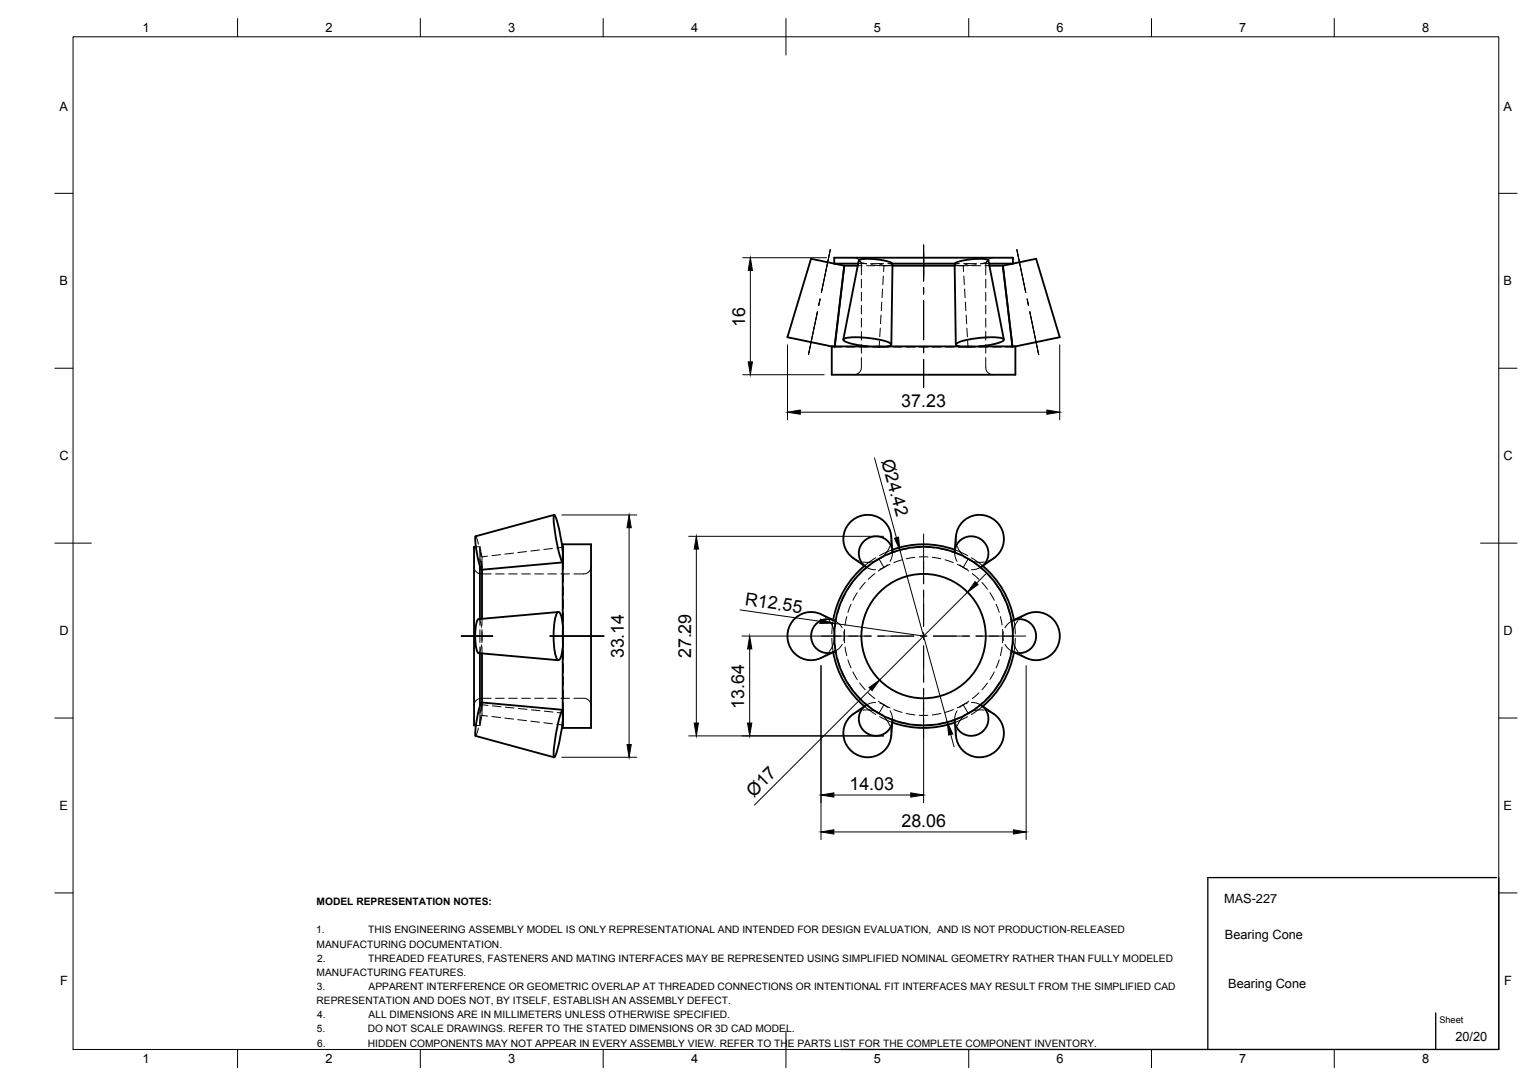
ISO-10303-21;
HEADER;
FILE_DESCRIPTION (('STEP AP214'),
    '1' );
FILE_NAME ( 'Bearing Cone.step', '2026-10-06T08:24:41', ( '' ), ( '' ), 'STEP AP214', 'Unspecified', '' );
FILE_SCHEMA (( 'AUTOMOTIVE_DESIGN' ));
ENDSEC;
DATA;
#68=CARTESIAN_POINT ( 'NONE',  ( 0.1516263115863346334, -0.2937912646890007973, 0.3972688187320929099 ) ) ;
#70=FACE_OUTER_BOUND ( 'NONE', #14571, .T. ) ;
#91=CYLINDRICAL_SURFACE ( 'NONE', #13414, 0.4941010236220472751 ) ;
#116=EDGE_LOOP ( 'NONE', ( #3270, #475, #22588, #2347 ) ) ;
#150=ADVANCED_FACE ( 'NONE', ( #5405 ), #14023, .T. ) ;
#166=CARTESIAN_POINT ( 'NONE',  ( 0.1490609433494345659, -0.2352065284464384953, -0.4168512521180542385 ) ) ;
#181=( BOUNDED_CURVE ( )  B_SPLINE_CURVE ( 3, ( #15130, #19634, #17231, #21476 ),
 .UNSPECIFIED., .F., .F. ) 
 B_SPLINE_CURVE_WITH_KNOTS ( ( 4, 4 ),
 ( 6.170019055269735375, 6.396351559089437089 ),
 .UNSPECIFIED. ) 
 CURVE ( )  GEOMETRIC_REPRESENTATION_ITEM ( )  RATIONAL_B_SPLINE_CURVE ( ( 1.000000000000000000, 0.9957356870045847019, 0.9957356870045847019, 1.000000000000000000 ) ) 
 REPRESENTATION_ITEM ( '' )  ) ;
#206=DIRECTION ( 'NONE',  ( 0.000000000000000000, 1.000000000000000000, 0.000000000000000000 ) ) ;
#228=ORIENTED_EDGE ( 'NONE', *, *, #21922, .T. ) ;
#246=CARTESIAN_POINT ( 'NONE',  ( 0.1490609433615242285, 0.4786070381542913421, 0.000000000000000000 ) ) ;
#280=VERTEX_POINT ( 'NONE', #5695 ) ;
#284=EDGE_CURVE ( 'NONE', #11054, #21365, #5605, .T. ) ;
#304=B_SPLINE_CURVE_WITH_KNOTS ( 'NONE', 3,
 ( #11360, #4990, #21548, #4455 ),
 .UNSPECIFIED., .F., .F.,
 ( 4, 4 ),
 ( 1.743059029969425078, 1.744705333033724992 ),
 .UNSPECIFIED. ) ;
#356=ADVANCED_FACE ( 'NONE', ( #15159 ), #8639, .T. ) ;
#373=EDGE_CURVE ( 'NONE', #24937, #5795, #15104, .T. ) ;
#380=EDGE_CURVE ( 'NONE', #22824, #12297, #25600, .T. ) ;
#390=AXIS2_PLACEMENT_3D ( 'NONE', #12393, #16488, #25245 ) ;
#413=ORIENTED_EDGE ( 'NONE', *, *, #20952, .T. ) ;
#463=ORIENTED_EDGE ( 'NONE', *, *, #26682, .F. ) ;
#468=CARTESIAN_POINT ( 'NONE',  ( 0.1525037638700916243, 0.2314035372547586233, -0.4381595109572587465 ) ) ;
#475=ORIENTED_EDGE ( 'NONE', *, *, #3137, .F. ) ;
#498=DIRECTION ( 'NONE',  ( 0.000000000000000000, 1.000000000000000000, 0.000000000000000000 ) ) ;
#503=LINE ( 'NONE', #20402, #13869 ) ;
#519=FACE_OUTER_BOUND ( 'NONE', #10794, .T. ) ;
#524=LINE ( 'NONE', #2219, #4201 ) ;
#525=CARTESIAN_POINT ( 'NONE',  ( 0.1490609433494345937, 0.2434005097105403082, -0.4121204548294903347 ) ) ;
#532=B_SPLINE_CURVE_WITH_KNOTS ( 'NONE', 3,
 ( #24989, #10725, #23173, #16808 ),
 .UNSPECIFIED., .F., .F.,
 ( 4, 4 ),
 ( 0.9895101543494979612, 0.9911564574137969874 ),
 .UNSPECIFIED. ) ;
#546=DIRECTION ( 'NONE',  ( 1.000000000000000000, 0.000000000000000000, 0.000000000000000000 ) ) ;
#558=DIRECTION ( 'NONE',  ( 1.000000000000000000, 0.000000000000000000, 0.000000000000000000 ) ) ;
#563=ORIENTED_EDGE ( 'NONE', *, *, #5290, .F. ) ;
#593=CARTESIAN_POINT ( 'NONE',  ( 0.2019525613798653918, -0.3664466487725785426, 0.6347042139374529102 ) ) ;
#615=EDGE_CURVE ( 'NONE', #12438, #5795, #14823, .T. ) ;
#627=EDGE_LOOP ( 'NONE', ( #9029, #26205 ) ) ;
#662=ORIENTED_EDGE ( 'NONE', *, *, #19173, .T. ) ;
#665=EDGE_CURVE ( 'NONE', #15651, #12947, #18212, .T. ) ;
#677=AXIS2_PLACEMENT_3D ( 'NONE', #5334, #26801, #20450 ) ;
#679=CARTESIAN_POINT ( 'NONE',  ( 0.1512834625131836974, 0.2028719039650156708, -0.4452748529150018508 ) ) ;
#688=FACE_OUTER_BOUND ( 'NONE', #8896, .T. ) ;
#707=DIRECTION ( 'NONE',  ( 1.000000000000000000, 0.000000000000000000, 0.000000000000000000 ) ) ;
#714=DIRECTION ( 'NONE',  ( -0.9575713608335526539, 0.1440981340193007720, -0.2495852893972995146 ) ) ;
#732=ORIENTED_EDGE ( 'NONE', *, *, #14585, .T. ) ;
#748=CARTESIAN_POINT ( 'NONE',  ( 0.1638952246732497953, 0.5499255957412874096, 0.000000000000000000 ) ) ;
#773=CARTESIAN_POINT ( 'NONE',  ( 0.1493402947442837025, 0.2231667116155127972, 0.4250100353273641440 ) ) ;
#781=DIRECTION ( 'NONE',  ( 0.000000000000000000, -0.8660254037844389297, -0.4999999999999994449 ) ) ;
#807=EDGE_CURVE ( 'NONE', #21046, #2655, #23735, .T. ) ;
#826=CIRCLE ( 'NONE', #11202, 0.1298643763538141760 ) ;
#843=DIRECTION ( 'NONE',  ( -0.9790454724845840673, 0.1018208755700876073, -0.1763589297585415050 ) ) ;
#872=ORIENTED_EDGE ( 'NONE', *, *, #24132, .F. ) ;
#873=AXIS2_PLACEMENT_3D ( 'NONE', #26941, #1100, #24946 ) ;
#898=DIRECTION ( 'NONE',  ( -0.9790454724845842893, -0.1018208755700884260, -0.1763589297585410332 ) ) ;
#904=( CONVERSION_BASED_UNIT ( 'INCH', #18242 ) LENGTH_UNIT ( ) NAMED_UNIT ( #24418 ) ) ;
#907=CARTESIAN_POINT ( 'NONE',  ( 0.6299212598425196763, -0.4807043897637795493, 5.886930922602943265E-17 ) ) ;
#915=CARTESIAN_POINT ( 'NONE',  ( 0.1755067523729419432, -0.3028750839302634112, 0.5245950337139047015 ) ) ;
#983=EDGE_LOOP ( 'NONE', ( #23970, #6463, #1289, #16251, #21520, #7050 ) ) ;
#984=CARTESIAN_POINT ( 'NONE',  ( 0.5869493968219645641, 0.2133897621573078718, 0.3696019098714952711 ) ) ;
#1004=CARTESIAN_POINT ( 'NONE',  ( 0.1490609433494345659, -0.4786070381568058862, -0.004730797288060355210 ) ) ;
#1011=VERTEX_POINT ( 'NONE', #5046 ) ;
#1060=DIRECTION ( 'NONE',  ( 1.000000000000000000, 0.000000000000000000, 0.000000000000000000 ) ) ;
#1100=DIRECTION ( 'NONE',  ( 0.9790454724845839563, -0.2036417511401769909, 0.000000000000000000 ) ) ;
#1114=AXIS2_PLACEMENT_3D ( 'NONE', #7079, #15697, #24300 ) ;
#1125=ORIENTED_EDGE ( 'NONE', *, *, #21190, .F. ) ;
#1130=CARTESIAN_POINT ( 'NONE',  ( 0.1516263115863346334, 0.4909405214979283838, 0.05579628926458630317 ) ) ;
#1146=CARTESIAN_POINT ( 'NONE',  ( 0.1512183756280983948, -0.4867863319339438277, -0.04701115990130280697 ) ) ;
#1151=DIRECTION ( 'NONE',  ( 0.000000000000000000, -1.000000000000000000, 0.000000000000000000 ) ) ;
#1158=CIRCLE ( 'NONE', #19655, 0.3740157480314960647 ) ;
#1186=EDGE_CURVE ( 'NONE', #12297, #1011, #18232, .T. ) ;
#1189=DIRECTION ( 'NONE',  ( -0.9790454724845842893, 0.2036417511401760472, 0.000000000000000000 ) ) ;
#1202=DIRECTION ( 'NONE',  ( 0.000000000000000000, 1.000000000000000000, 0.000000000000000000 ) ) ;
#1209=ORIENTED_EDGE ( 'NONE', *, *, #27427, .F. ) ;
#1231=VERTEX_POINT ( 'NONE', #23141 ) ;
#1241=CARTESIAN_POINT ( 'NONE',  ( 0.1516263115863346334, -0.1971492568089275588, -0.4530651079966787620 ) ) ;
#1262=CONICAL_SURFACE ( 'NONE', #22899, 0.4526932812344527379, 0.1178097243749990780 ) ;
#1265=ORIENTED_EDGE ( 'NONE', *, *, #26244, .T. ) ;
#1275=CARTESIAN_POINT ( 'NONE',  ( 0.1755067523729419432, 0.3028750839302634112, -0.5245950337139054787 ) ) ;
#1276=CIRCLE ( 'NONE', #19786, 0.3346456692913385988 ) ;
#1288=CARTESIAN_POINT ( 'NONE',  ( 0.1522836969735571200, 0.4941010236220468865, 0.01864847287710773294 ) ) ;
#1289=ORIENTED_EDGE ( 'NONE', *, *, #12310, .T. ) ;
#1294=AXIS2_PLACEMENT_3D ( 'NONE', #5908, #12769, #14538 ) ;
#1330=CARTESIAN_POINT ( 'NONE',  ( 0.1501355178992943573, -0.2698857342899688705, -0.4015219628616845671 ) ) ;
#1372=ORIENTED_EDGE ( 'NONE', *, *, #10616, .F. ) ;
#1455=DIRECTION ( 'NONE',  ( 1.000000000000000000, 0.000000000000000000, 0.000000000000000000 ) ) ;
#1592=CARTESIAN_POINT ( 'NONE',  ( 0.1516263115863346334, -0.4909405214979283838, 0.05579628926458630317 ) ) ;
#1605=DIRECTION ( 'NONE',  ( 1.000000000000000000, 0.000000000000000000, 0.000000000000000000 ) ) ;
#1606=B_SPLINE_CURVE_WITH_KNOTS ( 'NONE', 3,
 ( #13341, #17306, #19706, #24214 ),
 .UNSPECIFIED., .F., .F.,
 ( 4, 4 ),
 ( 1.743059029969425078, 1.744705333033724992 ),
 .UNSPECIFIED. ) ;
#1639=CARTESIAN_POINT ( 'NONE',  ( 0.6241887519799540485, -0.3029073140874564696, -0.5246508579836981490 ) ) ;
#1650=ORIENTED_EDGE ( 'NONE', *, *, #22521, .F. ) ;
#1658=DIRECTION ( 'NONE',  ( 0.000000000000000000, 0.000000000000000000, 1.000000000000000000 ) ) ;
#1670=ORIENTED_EDGE ( 'NONE', *, *, #22246, .T. ) ;
#1682=ORIENTED_EDGE ( 'NONE', *, *, #380, .T. ) ;
#1684=CARTESIAN_POINT ( 'NONE',  ( 0.1490609433537086470, -0.2477132731973591961, 0.4096304796931519165 ) ) ;
#1706=FACE_OUTER_BOUND ( 'NONE', #25350, .T. ) ;
#1707=AXIS2_PLACEMENT_3D ( 'NONE', #18329, #15682, #15955 ) ;
#1710=CIRCLE ( 'NONE', #390, 0.09143349766193344108 ) ;
#1722=ORIENTED_EDGE ( 'NONE', *, *, #4721, .T. ) ;
#1723=CARTESIAN_POINT ( 'NONE',  ( 0.1525037638700915965, -0.2314035372547590119, 0.4381595109572582469 ) ) ;
#1725=ORIENTED_EDGE ( 'NONE', *, *, #4241, .T. ) ;
#1752=ADVANCED_FACE ( 'NONE', ( #9783 ), #14715, .T. ) ;
#1760=EDGE_LOOP ( 'NONE', ( #17994, #18349, #7720, #19973 ) ) ;
#1761=CARTESIAN_POINT ( 'NONE',  ( 0.5925575908939920700, 0.000000000000000000, 0.000000000000000000 ) ) ;
#1791=CARTESIAN_POINT ( 'NONE',  ( 0.1490609433615242285, -0.4786070381542913421, 5.861244094488189820E-17 ) ) ;
#1802=VERTEX_POINT ( 'NONE', #20523 ) ;
#1810=ORIENTED_EDGE ( 'NONE', *, *, #27252, .F. ) ;
#1828=CARTESIAN_POINT ( 'NONE',  ( 0.03937007874015747977, 0.000000000000000000, -0.3740157480314960647 ) ) ;
#1832=DIRECTION ( 'NONE',  ( -0.9930684569432060016, -0.1175373975568611284, 1.439417707043116609E-17 ) ) ;
#1851=SURFACE_STYLE_FILL_AREA ( #5675 ) ;
#1889=EDGE_CURVE ( 'NONE', #18210, #12438, #181, .T. ) ;
#1893=CIRCLE ( 'NONE', #7287, 0.09143349766193344108 ) ;
#1908=AXIS2_PLACEMENT_3D ( 'NONE', #8443, #25400, #25959 ) ;
#1917=LINE ( 'NONE', #25369, #23538 ) ;
#1933=AXIS2_PLACEMENT_3D ( 'NONE', #3288, #11638, #1202 ) ;
#1998=DIRECTION ( 'NONE',  ( -0.9790454724845842893, -0.1018208755700880375, -0.1763589297585410332 ) ) ;
#2036=AXIS2_PLACEMENT_3D ( 'NONE', #3197, #18743, #11830 ) ;
#2068=EDGE_LOOP ( 'NONE', ( #14115, #15701, #8761 ) ) ;
#2072=ORIENTED_EDGE ( 'NONE', *, *, #18545, .F. ) ;
#2115=EDGE_CURVE ( 'NONE', #20796, #18835, #23260, .T. ) ;
#2127=ORIENTED_EDGE ( 'NONE', *, *, #27252, .T. ) ;
#2137=CARTESIAN_POINT ( 'NONE',  ( 0.6241887519799541595, 0.3029073140874564696, 0.5246508579836981490 ) ) ;
#2151=EDGE_LOOP ( 'NONE', ( #12416, #19888, #24371, #19139 ) ) ;
#2195=EDGE_CURVE ( 'NONE', #19740, #12947, #25112, .T. ) ;
#2202=DIRECTION ( 'NONE',  ( 0.000000000000000000, -1.000000000000000000, 0.000000000000000000 ) ) ;
#2205=EDGE_LOOP ( 'NONE', ( #5369, #6270, #18830, #662 ) ) ;
#2208=CARTESIAN_POINT ( 'NONE',  ( 0.3680051700917442714, -0.2263466406172265633, -0.3920438816715692831 ) ) ;
#2219=CARTESIAN_POINT ( 'NONE',  ( 0.5869493968219645641, -0.2133897621573078718, -0.3696019098714952711 ) ) ;
#2254=ORIENTED_EDGE ( 'NONE', *, *, #24577, .T. ) ;
#2256=CARTESIAN_POINT ( 'NONE',  ( 0.6241887519799541595, -0.6058146281749130502, 6.299353404003403643E-17 ) ) ;
#2264=ADVANCED_FACE ( 'NONE', ( #19133 ), #3370, .T. ) ;
#2270=CARTESIAN_POINT ( 'NONE',  ( 0.03937007874015747977, 0.000000000000000000, 0.000000000000000000 ) ) ;
#2278=EDGE_CURVE ( 'NONE', #15470, #23305, #13037, .T. ) ;
#2291=CARTESIAN_POINT ( 'NONE',  ( 0.3905379133858267737, 0.2805118110236220486, -0.4858607088160732390 ) ) ;
#2309=ORIENTED_EDGE ( 'NONE', *, *, #20542, .F. ) ;
#2347=ORIENTED_EDGE ( 'NONE', *, *, #4905, .T. ) ;
#2404=CARTESIAN_POINT ( 'NONE',  ( 0.1755067523729419432, -0.3028750839302637998, -0.5245950337139047015 ) ) ;
#2413=AXIS2_PLACEMENT_3D ( 'NONE', #22706, #7306, #5180 ) ;
#2417=ORIENTED_EDGE ( 'NONE', *, *, #4375, .T. ) ;
#2420=EDGE_LOOP ( 'NONE', ( #19438, #3974, #22960, #23219, #17211, #4913 ) ) ;
#2455=DIRECTION ( 'NONE',  ( 0.000000000000000000, 1.000000000000000000, 0.000000000000000000 ) ) ;
#2459=ORIENTED_EDGE ( 'NONE', *, *, #8343, .F. ) ;
#2510=AXIS2_PLACEMENT_3D ( 'NONE', #1761, #15064, #23256 ) ;
#2518=ADVANCED_FACE ( 'NONE', ( #17695 ), #26322, .T. ) ;
#2553=DIRECTION ( 'NONE',  ( -0.2036417511401758251, 0.9790454724845842893, -1.198984999999999602E-16 ) ) ;
#2558=CARTESIAN_POINT ( 'NONE',  ( 0.5869493968219645641, 0.2133897621573074832, -0.3696019098714952711 ) ) ;
#2560=CARTESIAN_POINT ( 'NONE',  ( 0.1525037638700915965, 0.2637554987713723320, -0.4194810972668293614 ) ) ;
#2593=CONICAL_SURFACE ( 'NONE', #18365, 0.4863540308881693086, 1.365720138124999927 ) ;
#2597=EDGE_CURVE ( 'NONE', #27102, #1802, #532, .T. ) ;
#2612=CIRCLE ( 'NONE', #6255, 0.4807043897637795493 ) ;
#2624=CARTESIAN_POINT ( 'NONE',  ( 0.1755067523729419432, -0.3028750839302634112, 0.5245950337139047015 ) ) ;
#2625=DIRECTION ( 'NONE',  ( -0.9790454724845842893, -0.2036417511401760472, 2.493892000000000781E-17 ) ) ;
#2629=VECTOR ( 'NONE', #24396, 39.37007874015748854 ) ;
#2634=EDGE_LOOP ( 'NONE', ( #21709, #12483, #8120, #17743, #16275, #6478 ) ) ;
#2644=CARTESIAN_POINT ( 'NONE',  ( 0.1638952246732497953, 0.2749627978706433162, -0.4762495361032464958 ) ) ;
#2655=VERTEX_POINT ( 'NONE', #1791 ) ;
#2664=LINE ( 'NONE', #17778, #15369 ) ;
#2697=ORIENTED_EDGE ( 'NONE', *, *, #12178, .T. ) ;
#2736=CARTESIAN_POINT ( 'NONE',  ( 0.1493472610806836076, 0.2566546340585424968, 0.4057060197093078080 ) ) ;
#2773=CARTESIAN_POINT ( 'NONE',  ( 0.1490609433615242285, 0.2393035190771452825, -0.4144858534716441278 ) ) ;
#2783=VECTOR ( 'NONE', #20849, 39.37007874015748854 ) ;
#2798=DIRECTION ( 'NONE',  ( -0.2036417511401761582, 0.4895227362422917006, -0.8478782506317886769 ) ) ;
#2800=CARTESIAN_POINT ( 'NONE',  ( 0.1516263115863346334, 0.4909405214979283838, 0.05579628926458630317 ) ) ;
#2815=CIRCLE ( 'NONE', #9598, 0.1298643763538142593 ) ;
#2816=EDGE_CURVE ( 'NONE', #23841, #11054, #503, .T. ) ;
#2818=CARTESIAN_POINT ( 'NONE',  ( 0.4130706566799093316, 0.3346769814300175616, 0.5796775359605756961 ) ) ;
#2821=FACE_OUTER_BOUND ( 'NONE', #2634, .T. ) ;
#2852=ORIENTED_EDGE ( 'NONE', *, *, #10985, .F. ) ;
#2861=DIRECTION ( 'NONE',  ( 0.000000000000000000, -1.000000000000000000, 0.000000000000000000 ) ) ;
#2863=DIRECTION ( 'NONE',  ( 0.000000000000000000, 1.000000000000000000, 0.000000000000000000 ) ) ;
#2893=CARTESIAN_POINT ( 'NONE',  ( 0.1516263115863346334, -0.4909405214979283838, -0.05579628926458622684 ) ) ;
#2912=ADVANCED_FACE ( 'NONE', ( #18261 ), #1262, .T. ) ;
#2942=ADVANCED_FACE ( 'NONE', ( #13763 ), #19849, .T. ) ;
#2964=AXIS2_PLACEMENT_3D ( 'NONE', #20804, #14767, #7960 ) ;
#2969=EDGE_CURVE ( 'NONE', #12210, #21566, #5764, .T. ) ;
#2982=AXIS2_PLACEMENT_3D ( 'NONE', #6922, #558, #9155 ) ;
#2988=DIRECTION ( 'NONE',  ( 1.000000000000000000, 0.000000000000000000, 0.000000000000000000 ) ) ;
#3015=DIRECTION ( 'NONE',  ( 0.2036417511401769631, -0.9790454724845838452, 1.198984999999999849E-16 ) ) ;
#3019=B_SPLINE_CURVE_WITH_KNOTS ( 'NONE', 3,
 ( #8186, #25271, #26975, #1130 ),
 .UNSPECIFIED., .F., .F.,
 ( 4, 4 ),
 ( 0.9893485554301200136, 0.9909948584944189287 ),
 .UNSPECIFIED. ) ;
#3048=FACE_OUTER_BOUND ( 'NONE', #23019, .T. ) ;
#3072=DIRECTION ( 'NONE',  ( -0.9790454724845842893, -0.1018208755700880375, 0.1763589297585410332 ) ) ;
#3137=EDGE_CURVE ( 'NONE', #21046, #13737, #4429, .T. ) ;
#3148=EDGE_LOOP ( 'NONE', ( #27180, #1682, #9509, #8478, #4115, #23919 ) ) ;
#3155=DIRECTION ( 'NONE',  ( -1.000000000000000000, 0.000000000000000000, 0.000000000000000000 ) ) ;
#3158=ORIENTED_EDGE ( 'NONE', *, *, #8802, .T. ) ;
#3164=CARTESIAN_POINT ( 'NONE',  ( 0.6055690743987126590, 0.2581485381169802973, 0.4471263839182408883 ) ) ;
#3170=EDGE_CURVE ( 'NONE', #22329, #8047, #3984, .T. ) ;
#3171=ORIENTED_EDGE ( 'NONE', *, *, #3875, .F. ) ;
#3187=CIRCLE ( 'NONE', #25763, 0.09143349766193348271 ) ;
#3197=CARTESIAN_POINT ( 'NONE',  ( 0.1506723201675407575, 0.000000000000000000, 0.000000000000000000 ) ) ;
#3203=CARTESIAN_POINT ( 'NONE',  ( 0.3149606299212598381, 0.3346456692913385988, 0.000000000000000000 ) ) ;
#3218=DIRECTION ( 'NONE',  ( -0.9790454724845842893, -0.1018208755700880375, 0.1763589297585410332 ) ) ;
#3219=VECTOR ( 'NONE', #21211, 39.37007874015748143 ) ;
#3228=ADVANCED_FACE ( 'NONE', ( #5573 ), #19299, .T. ) ;
#3250=CARTESIAN_POINT ( 'NONE',  ( 0.3905379133858267737, -0.2805118110236220486, 0.4858607088160724063 ) ) ;
#3263=CARTESIAN_POINT ( 'NONE',  ( 0.1522836969735571200, -0.4941010236220468865, 0.01864847287710767396 ) ) ;
#3266=DIRECTION ( 'NONE',  ( -0.2036417511401763802, 0.4895227362422922557, 0.8478782506317883438 ) ) ;
#3270=ORIENTED_EDGE ( 'NONE', *, *, #16719, .F. ) ;
#3283=CARTESIAN_POINT ( 'NONE',  ( 0.1504366439317612048, -0.2089021884548363517, 0.4380456861425212622 ) ) ;
#3286=DIRECTION ( 'NONE',  ( 1.000000000000000000, 0.000000000000000000, 0.000000000000000000 ) ) ;
#3288=CARTESIAN_POINT ( 'NONE',  ( 0.6299212598425196763, 0.4076750295275590741, 0.000000000000000000 ) ) ;
#3316=ORIENTED_EDGE ( 'NONE', *, *, #25771, .F. ) ;
#3331=DIRECTION ( 'NONE',  ( 1.000000000000000000, 0.000000000000000000, 0.000000000000000000 ) ) ;
#3335=ORIENTED_EDGE ( 'NONE', *, *, #7386, .T. ) ;
#3348=EDGE_LOOP ( 'NONE', ( #21676, #27774, #19131, #2459, #17124, #23248 ) ) ;
#3359=EDGE_CURVE ( 'NONE', #24341, #18758, #1276, .T. ) ;
#3370=CONICAL_SURFACE ( 'NONE', #2510, 0.4537419570391968415, 1.365720138124999927 ) ;
#3389=ORIENTED_EDGE ( 'NONE', *, *, #2969, .F. ) ;
#3402=CIRCLE ( 'NONE', #20119, 0.4807043897637795493 ) ;
#3427=DIRECTION ( 'NONE',  ( -0.9790454724845842893, 0.1018208755700882318, 0.1763589297585410332 ) ) ;
#3437=ORIENTED_EDGE ( 'NONE', *, *, #14859, .F. ) ;
#3485=ORIENTED_EDGE ( 'NONE', *, *, #3359, .T. ) ;
#3490=CARTESIAN_POINT ( 'NONE',  ( 0.1512834625133127053, -0.4870552862737996813, 0.04694520391073944698 ) ) ;
#3496=( GEOMETRIC_REPRESENTATION_CONTEXT ( 3 ) GLOBAL_UNCERTAINTY_ASSIGNED_CONTEXT ( ( #12494 ) ) GLOBAL_UNIT_ASSIGNED_CONTEXT ( ( #904, #22221, #26589 ) ) REPRESENTATION_CONTEXT ( 'NONE', 'WORKASPACE' ) ) ;
#3507=DIRECTION ( 'NONE',  ( 1.000000000000000000, 0.000000000000000000, 0.000000000000000000 ) ) ;
#3528=EDGE_CURVE ( 'NONE', #21046, #23841, #15047, .T. ) ;
#3641=EDGE_CURVE ( 'NONE', #23196, #17206, #10923, .T. ) ;
#3647=ORIENTED_EDGE ( 'NONE', *, *, #5093, .T. ) ;
#3707=ORIENTED_EDGE ( 'NONE', *, *, #4905, .F. ) ;
#3712=LINE ( 'NONE', #25184, #26502 ) ;
#3715=DIRECTION ( 'NONE',  ( 0.000000000000000000, 1.000000000000000000, 0.000000000000000000 ) ) ;
#3719=AXIS2_PLACEMENT_3D ( 'NONE', #15864, #10941, #19566 ) ;
#3721=CARTESIAN_POINT ( 'NONE',  ( 0.1516263115863346334, 0.4909405214979283838, -0.05579628926458630317 ) ) ;
#3752=VERTEX_POINT ( 'NONE', #11747 ) ;
#3795=ORIENTED_EDGE ( 'NONE', *, *, #16719, .T. ) ;
#3816=ORIENTED_EDGE ( 'NONE', *, *, #7420, .T. ) ;
#3875=EDGE_CURVE ( 'NONE', #5524, #15921, #14518, .T. ) ;
#3895=AXIS2_PLACEMENT_3D ( 'NONE', #12443, #1151, #14003 ) ;
#3901=AXIS2_PLACEMENT_3D ( 'NONE', #22366, #2988, #20243 ) ;
#3909=CARTESIAN_POINT ( 'NONE',  ( 0.1520645003680120011, -0.1970746732787106437, -0.4530975572029189435 ) ) ;
#3914=ORIENTED_EDGE ( 'NONE', *, *, #13598, .F. ) ;
#3926=ORIENTED_EDGE ( 'NONE', *, *, #25191, .F. ) ;
#3927=DIRECTION ( 'NONE',  ( -1.000000000000000000, 0.000000000000000000, 0.000000000000000000 ) ) ;
#3949=CARTESIAN_POINT ( 'NONE',  ( 0.1491281042588008532, -0.2312610231601890387, -0.4194211939771484432 ) ) ;
#3961=ORIENTED_EDGE ( 'NONE', *, *, #5628, .T. ) ;
#3964=EDGE_CURVE ( 'NONE', #19596, #7184, #4695, .T. ) ;
#3974=ORIENTED_EDGE ( 'NONE', *, *, #20018, .T. ) ;
#3984=CIRCLE ( 'NONE', #14349, 0.1298643763538141760 ) ;
#4037=CARTESIAN_POINT ( 'NONE',  ( 0.03937007874015747977, -0.3346456692913385988, 4.098227477461615257E-17 ) ) ;
#4053=CARTESIAN_POINT ( 'NONE',  ( 0.1516263115863346334, 0.2937912646890004087, -0.3972688187320929099 ) ) ;
#4068=ORIENTED_EDGE ( 'NONE', *, *, #20406, .T. ) ;
#4110=DIRECTION ( 'NONE',  ( -0.9790454724845842893, -0.1018208755700884260, -0.1763589297585410332 ) ) ;
#4115=ORIENTED_EDGE ( 'NONE', *, *, #9644, .F. ) ;
#4117=DIRECTION ( 'NONE',  ( -0.9790454724845839563, -0.2036417511401769909, 2.493892000000000165E-17 ) ) ;
#4130=EDGE_CURVE ( 'NONE', #4811, #25542, #26469, .T. ) ;
#4149=DIRECTION ( 'NONE',  ( 1.000000000000000000, 0.000000000000000000, 0.000000000000000000 ) ) ;
#4153=CARTESIAN_POINT ( 'NONE',  ( 0.1491281042588007977, 0.4788599204499175421, 0.009432676026079297657 ) ) ;
#4179=CONICAL_SURFACE ( 'NONE', #19499, 0.1106489370078740930, 0.08726646250000029414 ) ;
#4182=VERTEX_POINT ( 'NONE', #26651 ) ;
#4195=AXIS2_PLACEMENT_3D ( 'NONE', #18710, #5744, #7565 ) ;
#4201=VECTOR ( 'NONE', #6751, 39.37007874015748143 ) ;
#4213=FACE_OUTER_BOUND ( 'NONE', #20605, .T. ) ;
#4241=EDGE_CURVE ( 'NONE', #15651, #15443, #1710, .T. ) ;
#4268=CIRCLE ( 'NONE', #6503, 0.3346456692913385988 ) ;
#4308=CARTESIAN_POINT ( 'NONE',  ( 0.1520645003680120011, -0.2938566582910456804, 0.3972204521033409486 ) ) ;
#4336=CARTESIAN_POINT ( 'NONE',  ( 0.2019525613798653640, 0.7328932975451569742, 1.590379927979397374E-17 ) ) ;
#4340=DIRECTION ( 'NONE',  ( -0.1034422368825631960, 0.9946354626840587798, 0.000000000000000000 ) ) ;
#4375=EDGE_CURVE ( 'NONE', #13737, #23196, #11246, .T. ) ;
#4403=DIRECTION ( 'NONE',  ( -0.9790454724845842893, -0.1018208755700880375, -0.1763589297585410332 ) ) ;
#4429=CIRCLE ( 'NONE', #15696, 0.4267795243146149664 ) ;
#4433=( GEOMETRIC_REPRESENTATION_CONTEXT ( 3 ) GLOBAL_UNCERTAINTY_ASSIGNED_CONTEXT ( ( #12136 ) ) GLOBAL_UNIT_ASSIGNED_CONTEXT ( ( #10314, #27571, #18788 ) ) REPRESENTATION_CONTEXT ( 'NONE', 'WORKASPACE' ) ) ;
#4455=CARTESIAN_POINT ( 'NONE',  ( 0.1522836969735573143, -0.1970374587079578854, 0.4531137400369409374 ) ) ;
#4488=DIRECTION ( 'NONE',  ( -0.9790454724845842893, -0.1018208755700880375, 0.1763589297585410332 ) ) ;
#4502=CONICAL_SURFACE ( 'NONE', #26570, 0.4863540308881693086, 1.365720138124999927 ) ;
#4518=CIRCLE ( 'NONE', #9910, 0.1298643763538142593 ) ;
#4526=VERTEX_POINT ( 'NONE', #17471 ) ;
#4530=CONICAL_SURFACE ( 'NONE', #18538, 0.4526932812344527379, 0.1178097243749990780 ) ;
#4532=DIRECTION ( 'NONE',  ( -0.9790454724845842893, -0.2036417511401760472, 2.493892000000000781E-17 ) ) ;
#4557=DIRECTION ( 'NONE',  ( -0.2036417511401762415, -0.4895227362422910344, 0.8478782506317890100 ) ) ;
#4559=EDGE_CURVE ( 'NONE', #23196, #13737, #16668, .T. ) ;
#4570=FACE_OUTER_BOUND ( 'NONE', #17854, .T. ) ;
#4576=CARTESIAN_POINT ( 'NONE',  ( 0.3680051700917441604, 0.000000000000000000, 0.000000000000000000 ) ) ;
#4584=DIRECTION ( 'NONE',  ( 0.000000000000000000, 1.000000000000000000, 0.000000000000000000 ) ) ;
#4594=ORIENTED_EDGE ( 'NONE', *, *, #14859, .T. ) ;
#4607=CARTESIAN_POINT ( 'NONE',  ( 0.1522836969735573143, 0.2938892803217901806, -0.3971963147566898167 ) ) ;
#4659=LINE ( 'NONE', #15145, #3219 ) ;
#4695=LINE ( 'NONE', #15721, #11225 ) ;
#4710=AXIS2_PLACEMENT_3D ( 'NONE', #8153, #20999, #16762 ) ;
#4721=EDGE_CURVE ( 'NONE', #15921, #17206, #826, .T. ) ;
#4723=CARTESIAN_POINT ( 'NONE',  ( 0.3680051700917441604, 0.000000000000000000, 0.000000000000000000 ) ) ;
#4731=ORIENTED_EDGE ( 'NONE', *, *, #2278, .T. ) ;
#4747=ORIENTED_EDGE ( 'NONE', *, *, #3170, .F. ) ;
#4752=VERTEX_POINT ( 'NONE', #15014 ) ;
#4762=CARTESIAN_POINT ( 'NONE',  ( 0.1504127680535784495, -0.2090906986543966672, -0.4378338296930543438 ) ) ;
#4773=VERTEX_POINT ( 'NONE', #6251 ) ;
#4776=ADVANCED_FACE ( 'NONE', ( #70 ), #12569, .T. ) ;
#4782=ORIENTED_EDGE ( 'NONE', *, *, #16080, .T. ) ;
#4811=VERTEX_POINT ( 'NONE', #7588 ) ;
#4814=CARTESIAN_POINT ( 'NONE',  ( 0.1516263115863346334, -0.1971492568089275588, -0.4530651079966787620 ) ) ;
#4833=DIRECTION ( 'NONE',  ( 1.000000000000000000, 0.000000000000000000, 0.000000000000000000 ) ) ;
#4842=DIRECTION ( 'NONE',  ( 0.000000000000000000, 1.000000000000000000, 0.000000000000000000 ) ) ;
#4872=ORIENTED_EDGE ( 'NONE', *, *, #3528, .T. ) ;
#4905=EDGE_CURVE ( 'NONE', #2655, #11023, #16180, .T. ) ;
#4913=ORIENTED_EDGE ( 'NONE', *, *, #807, .F. ) ;
#4919=CARTESIAN_POINT ( 'NONE',  ( 0.1518453844022533417, -0.4909359254662000183, 0.05583672883938764486 ) ) ;
#4980=DIRECTION ( 'NONE',  ( 0.000000000000000000, -1.000000000000000000, 0.000000000000000000 ) ) ;
#4988=ORIENTED_EDGE ( 'NONE', *, *, #27217, .F. ) ;
#4990=CARTESIAN_POINT ( 'NONE',  ( 0.1518453844022533417, -0.1971119370939669324, 0.4530813475038464877 ) ) ;
#5003=CARTESIAN_POINT ( 'NONE',  ( 0.5925575908939920700, 0.000000000000000000, 0.000000000000000000 ) ) ;
#5015=DIRECTION ( 'NONE',  ( 0.000000000000000000, -1.000000000000000000, 0.000000000000000000 ) ) ;
#5019=ORIENTED_EDGE ( 'NONE', *, *, #23730, .F. ) ;
#5027=EDGE_LOOP ( 'NONE', ( #9275, #3316, #17408, #8169 ) ) ;
#5034=AXIS2_PLACEMENT_3D ( 'NONE', #5818, #27283, #27147 ) ;
#5046=CARTESIAN_POINT ( 'NONE',  ( 0.1516263115863346334, 0.4909405214979283838, -0.05579628926458630317 ) ) ;
#5074=CARTESIAN_POINT ( 'NONE',  ( 0.6299212598425196763, 0.000000000000000000, -0.3740157480314960647 ) ) ;
#5093=EDGE_CURVE ( 'NONE', #13737, #15651, #22932, .T. ) ;
#5097=CARTESIAN_POINT ( 'NONE',  ( 0.5925575908939920700, 0.000000000000000000, 0.000000000000000000 ) ) ;
#5131=CARTESIAN_POINT ( 'NONE',  ( 0.1504231045792249755, 0.2090266774008008310, 0.4379142800569870153 ) ) ;
#5133=CARTESIAN_POINT ( 'NONE',  ( 0.5869493968219645641, 0.000000000000000000, 0.000000000000000000 ) ) ;
#5136=CARTESIAN_POINT ( 'NONE',  ( 0.5925575908939920700, 0.2268709785195984208, -0.3929520615588126264 ) ) ;
#5148=CARTESIAN_POINT ( 'NONE',  ( 0.5869493968219645641, -0.4267795243146149664, 5.226543307086613929E-17 ) ) ;
#5155=ORIENTED_EDGE ( 'NONE', *, *, #19745, .T. ) ;
#5159=ORIENTED_EDGE ( 'NONE', *, *, #26948, .F. ) ;
#5169=CIRCLE ( 'NONE', #26382, 0.3346456692913385988 ) ;
#5180=DIRECTION ( 'NONE',  ( 0.000000000000000000, 1.000000000000000000, 0.000000000000000000 ) ) ;
#5231=EDGE_LOOP ( 'NONE', ( #10752, #21180, #5159, #27091 ) ) ;
#5278=DIRECTION ( 'NONE',  ( -0.9790454724845842893, -0.1018208755700880375, 0.1763589297585410332 ) ) ;
#5290=EDGE_CURVE ( 'NONE', #8047, #17815, #15314, .T. ) ;
#5334=CARTESIAN_POINT ( 'NONE',  ( 0.1755067523729419432, 0.6057501678605275997, 0.000000000000000000 ) ) ;
#5354=DIRECTION ( 'NONE',  ( -0.2036417511401758251, 0.4895227362422921447, -0.8478782506317885659 ) ) ;
#5369=ORIENTED_EDGE ( 'NONE', *, *, #24366, .T. ) ;
#5382=AXIS2_PLACEMENT_3D ( 'NONE', #3250, #26145, #11165 ) ;
#5405=FACE_OUTER_BOUND ( 'NONE', #5739, .T. ) ;
#5407=CARTESIAN_POINT ( 'NONE',  ( 0.1490609433615240342, 0.2393035190771456711, 0.4144858534716441278 ) ) ;
#5427=CARTESIAN_POINT ( 'NONE',  ( 0.1504778549385457909, -0.2746646418458098537, -0.4002635090060460699 ) ) ;
#5438=ORIENTED_EDGE ( 'NONE', *, *, #9660, .T. ) ;
#5465=EDGE_CURVE ( 'NONE', #280, #9781, #24261, .T. ) ;
#5494=CARTESIAN_POINT ( 'NONE',  ( 0.1522836969735573143, -0.4909267390297480382, 0.05591742528025181458 ) ) ;
#5497=CIRCLE ( 'NONE', #5034, 0.4786070381542913421 ) ;
#5522=EDGE_CURVE ( 'NONE', #26797, #21888, #18883, .T. ) ;
#5524=VERTEX_POINT ( 'NONE', #22146 ) ;
#5528=CARTESIAN_POINT ( 'NONE',  ( 0.6299212598425196763, 0.000000000000000000, 0.000000000000000000 ) ) ;
#5533=CARTESIAN_POINT ( 'NONE',  ( 0.6299212598425196763, 0.4807043897637795493, 0.000000000000000000 ) ) ;
#5541=CONICAL_SURFACE ( 'NONE', #13632, 0.1106489370078740098, 0.08726646250000029414 ) ;
#5565=CARTESIAN_POINT ( 'NONE',  ( 0.5869493968219645641, -0.4267795243146149664, 5.226543307086613929E-17 ) ) ;
#5571=ORIENTED_EDGE ( 'NONE', *, *, #25191, .T. ) ;
#5573=FACE_OUTER_BOUND ( 'NONE', #14108, .T. ) ;
#5605=CIRCLE ( 'NONE', #7384, 0.4807043897637795493 ) ;
#5628=EDGE_CURVE ( 'NONE', #12967, #12297, #22501, .T. ) ;
#5675=FILL_AREA_STYLE ('',( #23053 ) ) ;
#5695=CARTESIAN_POINT ( 'NONE',  ( 0.5869493968219645641, 0.2133897621573074832, 0.3696019098714952711 ) ) ;
#5715=DIRECTION ( 'NONE',  ( -0.9930684569549264040, -0.1175373974578370340, 1.439418000000000363E-17 ) ) ;
#5739=EDGE_LOOP ( 'NONE', ( #21715, #3961, #23435, #27138 ) ) ;
#5744=DIRECTION ( 'NONE',  ( 1.000000000000000000, 0.000000000000000000, 0.000000000000000000 ) ) ;
#5764=CIRCLE ( 'NONE', #27414, 0.4941010236220472751 ) ;
#5795=VERTEX_POINT ( 'NONE', #17226 ) ;
#5814=ORIENTED_EDGE ( 'NONE', *, *, #13838, .F. ) ;
#5818=CARTESIAN_POINT ( 'NONE',  ( 0.1490609433615242285, 0.000000000000000000, 0.000000000000000000 ) ) ;
#5821=DIRECTION ( 'NONE',  ( -0.2036417511401769631, 0.9790454724845838452, 0.000000000000000000 ) ) ;
#5842=EDGE_LOOP ( 'NONE', ( #12784, #5438, #8571, #10405, #10856, #2127 ) ) ;
#5846=CARTESIAN_POINT ( 'NONE',  ( 0.4130706566799093316, -0.6693539628600351232, 6.842164547144469713E-17 ) ) ;
#5869=ORIENTED_EDGE ( 'NONE', *, *, #27217, .T. ) ;
#5894=ORIENTED_EDGE ( 'NONE', *, *, #21466, .F. ) ;
#5908=CARTESIAN_POINT ( 'NONE',  ( 0.1755067523729419432, 0.6057501678605275997, 0.000000000000000000 ) ) ;
#5910=LINE ( 'NONE', #12669, #19441 ) ;
#5911=CARTESIAN_POINT ( 'NONE',  ( 0.1495939273659978308, -0.4806208190371700772, -0.02345246241341144428 ) ) ;
#5953=ORIENTED_EDGE ( 'NONE', *, *, #10677, .T. ) ;
#5979=ORIENTED_EDGE ( 'NONE', *, *, #22943, .T. ) ;
#5982=EDGE_LOOP ( 'NONE', ( #19905, #19422 ) ) ;
#6002=CIRCLE ( 'NONE', #23600, 0.09143349766193348271 ) ;
#6008=ORIENTED_EDGE ( 'NONE', *, *, #8644, .T. ) ;
#6040=ADVANCED_FACE ( 'NONE', ( #13170 ), #15592, .T. ) ;
#6041=DIRECTION ( 'NONE',  ( 1.000000000000000000, 0.000000000000000000, 0.000000000000000000 ) ) ;
#6052=CIRCLE ( 'NONE', #20937, 0.03937007874015744507 ) ;
#6056=CARTESIAN_POINT ( 'NONE',  ( 0.1490609433615242285, -0.4786070381542913421, 5.861244094488189820E-17 ) ) ;
#6062=CARTESIAN_POINT ( 'NONE',  ( 0.6241887519799541595, 0.6058146281749130502, 1.119737402735601890E-17 ) ) ;
#6097=ADVANCED_FACE ( 'NONE', ( #15995 ), #12610, .T. ) ;
#6099=B_SPLINE_CURVE_WITH_KNOTS ( 'NONE', 3,
 ( #10720, #166, #3949, #19194, #8332, #4762, #9402, #19753 ),
 .UNSPECIFIED., .F., .F.,
 ( 4, 2, 2, 4 ),
 ( 0.000000000000000000, 0.2500000000000000000, 0.5000000000000000000, 1.000000000000000000 ),
 .UNSPECIFIED. ) ;
#6115=AXIS2_PLACEMENT_3D ( 'NONE', #23276, #21425, #10395 ) ;
#6147=ORIENTED_EDGE ( 'NONE', *, *, #25869, .T. ) ;
#6153=CARTESIAN_POINT ( 'NONE',  ( 0.5869493968219645641, -0.4267795243146149664, 5.226543307086613929E-17 ) ) ;
#6180=AXIS2_PLACEMENT_3D ( 'NONE', #11911, #1189, #9789 ) ;
#6210=DIRECTION ( 'NONE',  ( 0.000000000000000000, 1.000000000000000000, 0.000000000000000000 ) ) ;
#6238=ORIENTED_EDGE ( 'NONE', *, *, #14772, .F. ) ;
#6243=ADVANCED_FACE ( 'NONE', ( #25092 ), #14380, .T. ) ;
#6251=CARTESIAN_POINT ( 'NONE',  ( 0.5905511811023621549, 0.3346456692913385988, 0.000000000000000000 ) ) ;
#6255=AXIS2_PLACEMENT_3D ( 'NONE', #5528, #14149, #16527 ) ;
#6270=ORIENTED_EDGE ( 'NONE', *, *, #20896, .F. ) ;
#6288=ORIENTED_EDGE ( 'NONE', *, *, #2195, .F. ) ;
#6331=CARTESIAN_POINT ( 'NONE',  ( 0.3680051700917441604, 0.000000000000000000, 0.000000000000000000 ) ) ;
#6354=EDGE_CURVE ( 'NONE', #12205, #18210, #25077, .T. ) ;
#6398=EDGE_LOOP ( 'NONE', ( #12982, #3707, #22746, #3158 ) ) ;
#6436=ORIENTED_EDGE ( 'NONE', *, *, #12114, .T. ) ;
#6463=ORIENTED_EDGE ( 'NONE', *, *, #23730, .T. ) ;
#6471=EDGE_CURVE ( 'NONE', #5795, #7963, #13561, .T. ) ;
#6478=ORIENTED_EDGE ( 'NONE', *, *, #284, .F. ) ;
#6503=AXIS2_PLACEMENT_3D ( 'NONE', #8376, #23771, #8641 ) ;
#6544=DIRECTION ( 'NONE',  ( 0.2036417511401769909, 0.4895227362422910344, -0.8478782506317890100 ) ) ;
#6580=CARTESIAN_POINT ( 'NONE',  ( 0.1520645003235147619, -0.2938566582844236441, -0.3972204521082409734 ) ) ;
#6598=CARTESIAN_POINT ( 'NONE',  ( 0.1522836969815822838, 0.1970374587168192970, 0.4531137400420984229 ) ) ;
#6617=( BOUNDED_CURVE ( )  B_SPLINE_CURVE ( 3, ( #20818, #21632, #27326, #3721 ),
 .UNSPECIFIED., .F., .F. ) 
 B_SPLINE_CURVE_WITH_KNOTS ( ( 4, 4 ),
 ( 0.000000000000000000, 0.1131662519098511482 ),
 .UNSPECIFIED. ) 
 CURVE ( )  GEOMETRIC_REPRESENTATION_ITEM ( )  RATIONAL_B_SPLINE_CURVE ( ( 1.000000000000000000, 0.9989330679932157953, 0.9989330679932157953, 1.000000000000000000 ) ) 
 REPRESENTATION_ITEM ( '' )  ) ;
#6659=AXIS2_PLACEMENT_3D ( 'NONE', #3164, #7146, #24640 ) ;
#6660=CARTESIAN_POINT ( 'NONE',  ( 0.3905379133858267737, -0.5610236220472440971, 6.870559055118111198E-17 ) ) ;
#6662=DIRECTION ( 'NONE',  ( -0.9790454724845842893, 0.2036417511401760472, 0.000000000000000000 ) ) ;
#6665=DIRECTION ( 'NONE',  ( -0.2036417511401760472, 0.4895227362422920336, 0.8478782506317883438 ) ) ;
#6674=CIRCLE ( 'NONE', #22447, 0.1298643763538142593 ) ;
#6676=ORIENTED_EDGE ( 'NONE', *, *, #17110, .T. ) ;
#6718=DIRECTION ( 'NONE',  ( 1.000000000000000000, 0.000000000000000000, 0.000000000000000000 ) ) ;
#6742=EDGE_CURVE ( 'NONE', #21566, #19740, #22323, .T. ) ;
#6751=DIRECTION ( 'NONE',  ( 0.2036417511401759084, -0.4895227362422918116, -0.8478782506317885659 ) ) ;
#6752=CARTESIAN_POINT ( 'NONE',  ( 0.1504127680536208045, 0.2746298698235986602, -0.3999947715762637301 ) ) ;
#6773=DIRECTION ( 'NONE',  ( 0.000000000000000000, -1.000000000000000000, 0.000000000000000000 ) ) ;
#6811=VERTEX_POINT ( 'NONE', #26401 ) ;
#6885=ORIENTED_EDGE ( 'NONE', *, *, #3641, .T. ) ;
#6922=CARTESIAN_POINT ( 'NONE',  ( 0.1522836969735573143, 0.000000000000000000, 0.000000000000000000 ) ) ;
#6931=EDGE_CURVE ( 'NONE', #26797, #26980, #23457, .T. ) ;
#6974=ORIENTED_EDGE ( 'NONE', *, *, #3528, .F. ) ;
#6985=DIRECTION ( 'NONE',  ( 1.000000000000000000, 0.000000000000000000, 0.000000000000000000 ) ) ;
#6986=CONICAL_SURFACE ( 'NONE', #4710, 0.1106489370078740930, 0.08726646250000029414 ) ;
#6990=ORIENTED_EDGE ( 'NONE', *, *, #16984, .T. ) ;
#7008=EDGE_LOOP ( 'NONE', ( #11460, #1209, #6288, #16790 ) ) ;
#7025=VECTOR ( 'NONE', #13303, 39.37007874015748854 ) ;
#7038=CARTESIAN_POINT ( 'NONE',  ( 0.1501355178992943573, 0.2127853528708066044, -0.4344888834448818460 ) ) ;
#7050=ORIENTED_EDGE ( 'NONE', *, *, #1186, .F. ) ;
#7053=B_SPLINE_CURVE_WITH_KNOTS ( 'NONE', 3,
 ( #5494, #16497, #3490, #18604, #10136, #27245, #10274, #14262 ),
 .UNSPECIFIED., .F., .F.,
 ( 4, 2, 2, 4 ),
 ( 0.000000000000000000, 0.2500000000000000000, 0.5000000000000000000, 1.000000000000000000 ),
 .UNSPECIFIED. ) ;
#7059=EDGE_LOOP ( 'NONE', ( #3335, #3816, #12558, #872, #3485 ) ) ;
#7079=CARTESIAN_POINT ( 'NONE',  ( 0.5869493968219645641, 0.000000000000000000, 0.000000000000000000 ) ) ;
#7086=ORIENTED_EDGE ( 'NONE', *, *, #2115, .F. ) ;
#7098=DIRECTION ( 'NONE',  ( 1.000000000000000000, 0.000000000000000000, 0.000000000000000000 ) ) ;
#7105=DIRECTION ( 'NONE',  ( 0.000000000000000000, 1.000000000000000000, 0.000000000000000000 ) ) ;
#7130=DIRECTION ( 'NONE',  ( 0.000000000000000000, 1.000000000000000000, 0.000000000000000000 ) ) ;
#7131=CARTESIAN_POINT ( 'NONE',  ( 0.1490609433537086470, 0.2477131595981420797, 0.4096305452796897839 ) ) ;
#7133=ORIENTED_EDGE ( 'NONE', *, *, #18122, .T. ) ;
#7146=DIRECTION ( 'NONE',  ( -0.9790454724845842893, 0.1018208755700880375, 0.1763589297585410332 ) ) ;
#7184=VERTEX_POINT ( 'NONE', #21594 ) ;
#7193=FACE_OUTER_BOUND ( 'NONE', #20077, .T. ) ;
#7210=EDGE_LOOP ( 'NONE', ( #10542, #1722, #26476 ) ) ;
#7214=CARTESIAN_POINT ( 'NONE',  ( 0.5981657849660177995, 0.000000000000000000, 0.000000000000000000 ) ) ;
#7239=CARTESIAN_POINT ( 'NONE',  ( 0.3905379133858267737, -0.2805118110236220486, -0.4858607088160724063 ) ) ;
#7254=CARTESIAN_POINT ( 'NONE',  ( 0.1490609433537086470, -0.2308938785792120918, 0.4193411617035458505 ) ) ;
#7260=DIRECTION ( 'NONE',  ( -0.2036417511401761582, -0.4895227362422917006, -0.8478782506317886769 ) ) ;
#7287=AXIS2_PLACEMENT_3D ( 'NONE', #21523, #8657, #17280 ) ;
#7306=DIRECTION ( 'NONE',  ( -1.000000000000000000, 0.000000000000000000, 0.000000000000000000 ) ) ;
#7321=CARTESIAN_POINT ( 'NONE',  ( 0.03937007874015747977, 0.3346456692913385988, 0.000000000000000000 ) ) ;
#7332=CARTESIAN_POINT ( 'NONE',  ( 0.6055690743987126590, -0.2581485381169802973, 0.4471263839182408883 ) ) ;
#7384=AXIS2_PLACEMENT_3D ( 'NONE', #10051, #16551, #7808 ) ;
#7386=EDGE_CURVE ( 'NONE', #18758, #1231, #23938, .T. ) ;
#7387=FACE_OUTER_BOUND ( 'NONE', #983, .T. ) ;
#7413=DIRECTION ( 'NONE',  ( -0.2036417511401758251, -0.9790454724845842893, 0.000000000000000000 ) ) ;
#7415=ORIENTED_EDGE ( 'NONE', *, *, #22856, .T. ) ;
#7420=EDGE_CURVE ( 'NONE', #1231, #4752, #12190, .T. ) ;
#7439=PLANE ( 'NONE',  #25438 ) ;
#7444=DIRECTION ( 'NONE',  ( 0.000000000000000000, 0.000000000000000000, -1.000000000000000000 ) ) ;
#7450=CARTESIAN_POINT ( 'NONE',  ( 0.3680051700917442714, 0.2263466406172266743, -0.3920438816715699493 ) ) ;
#7484=CARTESIAN_POINT ( 'NONE',  ( 0.1522836969735573143, 0.4909267390297480382, -0.05591742528025173131 ) ) ;
#7492=VERTEX_POINT ( 'NONE', #16612 ) ;
#7512=ORIENTED_EDGE ( 'NONE', *, *, #6931, .F. ) ;
#7518=DIRECTION ( 'NONE',  ( 1.000000000000000000, 0.000000000000000000, 0.000000000000000000 ) ) ;
#7519=AXIS2_PLACEMENT_3D ( 'NONE', #23815, #6718, #4584 ) ;
#7532=CYLINDRICAL_SURFACE ( 'NONE', #3901, 0.3346456692913385988 ) ;
#7545=DIRECTION ( 'NONE',  ( 1.000000000000000000, 0.000000000000000000, 0.000000000000000000 ) ) ;
#7553=AXIS2_PLACEMENT_3D ( 'NONE', #10459, #4117, #5821 ) ;
#7554=PRODUCT_CONTEXT ( 'NONE', #24400, 'mechanical' ) ;
#7565=DIRECTION ( 'NONE',  ( 0.000000000000000000, 1.000000000000000000, 0.000000000000000000 ) ) ;
#7572=ORIENTED_EDGE ( 'NONE', *, *, #807, .T. ) ;
#7588=CARTESIAN_POINT ( 'NONE',  ( 0.1522836969735573143, 0.1970374587079574968, -0.4531137400369417145 ) ) ;
#7607=DIRECTION ( 'NONE',  ( 0.000000000000000000, 1.224646799147353700E-16, 1.000000000000000000 ) ) ;
#7633=DIRECTION ( 'NONE',  ( 1.000000000000000000, 0.000000000000000000, 0.000000000000000000 ) ) ;
#7638=CARTESIAN_POINT ( 'NONE',  ( 0.5869493968219645641, 0.2133897621573070669, -0.3696019098714952711 ) ) ;
#7648=CARTESIAN_POINT ( 'NONE',  ( 0.6140435224042697371, 0.000000000000000000, 0.000000000000000000 ) ) ;
#7671=CARTESIAN_POINT ( 'NONE',  ( 0.1520643344662694629, -0.4930463976998556430, 0.03726710077533004067 ) ) ;
#7690=CARTESIAN_POINT ( 'NONE',  ( 0.1493472610806836354, -0.2230244025072592728, 0.4251224429483507206 ) ) ;
#7709=ORIENTED_EDGE ( 'NONE', *, *, #19745, .F. ) ;
#7720=ORIENTED_EDGE ( 'NONE', *, *, #22320, .F. ) ;
#7775=DIRECTION ( 'NONE',  ( 0.000000000000000000, -1.000000000000000000, 0.000000000000000000 ) ) ;
#7777=DIRECTION ( 'NONE',  ( -0.2036417511401760472, -0.4895227362422912565, 0.8478782506317888989 ) ) ;
#7795=CARTESIAN_POINT ( 'NONE',  ( 0.1522836969735573143, 0.000000000000000000, 0.000000000000000000 ) ) ;
#7808=DIRECTION ( 'NONE',  ( 0.000000000000000000, 1.000000000000000000, 0.000000000000000000 ) ) ;
#7822=CIRCLE ( 'NONE', #15061, 0.4807043897637795493 ) ;
#7825=TOROIDAL_SURFACE ( 'NONE', #23183, 0.3740157480314960647, 0.03937007874015747977 ) ;
#7839=CARTESIAN_POINT ( 'NONE',  ( 0.1512183756281006430, 0.4867863319339526540, 0.04701115990132218730 ) ) ;
#7925=AXIS2_PLACEMENT_3D ( 'NONE', #7239, #898, #3266 ) ;
#7934=AXIS2_PLACEMENT_3D ( 'NONE', #21928, #17544, #2553 ) ;
#7960=DIRECTION ( 'NONE',  ( 0.000000000000000000, 1.000000000000000000, 0.000000000000000000 ) ) ;
#7963=VERTEX_POINT ( 'NONE', #27321 ) ;
#7975=CARTESIAN_POINT ( 'NONE',  ( 0.1516263115863346334, -0.2937912646890007973, -0.3972688187320929099 ) ) ;
#7993=EDGE_LOOP ( 'NONE', ( #27242, #1265, #14498, #9901, #17346, #8002 ) ) ;
#8002=ORIENTED_EDGE ( 'NONE', *, *, #16984, .F. ) ;
#8047=VERTEX_POINT ( 'NONE', #20678 ) ;
#8049=MECHANICAL_DESIGN_GEOMETRIC_PRESENTATION_REPRESENTATION('',(#15273),#4433);
#8057=AXIS2_PLACEMENT_3D ( 'NONE', #6660, #4532, #19650 ) ;
#8062=AXIS2_PLACEMENT_3D ( 'NONE', #2270, #13144, #21359 ) ;
#8076=ADVANCED_FACE ( 'NONE', ( #14198 ), #9512, .F. ) ;
#8107=DIRECTION ( 'NONE',  ( 0.2036417511401769909, -0.4895227362422910344, 0.8478782506317890100 ) ) ;
#8120=ORIENTED_EDGE ( 'NONE', *, *, #27089, .T. ) ;
#8131=EDGE_CURVE ( 'NONE', #21888, #26797, #16759, .T. ) ;
#8140=ORIENTED_EDGE ( 'NONE', *, *, #22856, .F. ) ;
#8144=CARTESIAN_POINT ( 'NONE',  ( 0.1490609433615240342, -0.2393035190771456711, 0.4144858534716441278 ) ) ;
#8153=CARTESIAN_POINT ( 'NONE',  ( 0.3905379133858267737, 0.2805118110236220486, 0.4858607088160724063 ) ) ;
#8169=ORIENTED_EDGE ( 'NONE', *, *, #373, .T. ) ;
#8172=ORIENTED_EDGE ( 'NONE', *, *, #8358, .F. ) ;
#8182=VECTOR ( 'NONE', #20130, 39.37007874015748854 ) ;
#8186=CARTESIAN_POINT ( 'NONE',  ( 0.1522836969735573143, 0.4909267390297480382, 0.05591742528025173131 ) ) ;
#8203=CARTESIAN_POINT ( 'NONE',  ( 0.6241887519799542705, 0.3029073140874565251, -0.5246508579836989261 ) ) ;
#8231=CARTESIAN_POINT ( 'NONE',  ( 0.1516263115863346334, -0.1971492568089271424, 0.4530651079966787620 ) ) ;
#8260=EDGE_CURVE ( 'NONE', #17635, #4182, #8805, .T. ) ;
#8293=CARTESIAN_POINT ( 'NONE',  ( 0.1518453843511950729, 0.1971119371026649747, 0.4530813475000622370 ) ) ;
#8332=CARTESIAN_POINT ( 'NONE',  ( 0.1495939273659548374, -0.2199999812874746663, -0.4279560700802453321 ) ) ;
#8337=DIRECTION ( 'NONE',  ( 0.000000000000000000, 0.000000000000000000, -1.000000000000000000 ) ) ;
#8343=EDGE_CURVE ( 'NONE', #4773, #12691, #18062, .T. ) ;
#8358=EDGE_CURVE ( 'NONE', #17275, #12205, #15228, .T. ) ;
#8376=CARTESIAN_POINT ( 'NONE',  ( 0.5905511811023621549, 0.000000000000000000, 0.000000000000000000 ) ) ;
#8382=AXIS2_PLACEMENT_3D ( 'NONE', #24697, #7545, #16174 ) ;
#8388=EDGE_CURVE ( 'NONE', #21046, #2655, #25189, .T. ) ;
#8443=CARTESIAN_POINT ( 'NONE',  ( 0.3149606299212598381, 0.000000000000000000, 0.000000000000000000 ) ) ;
#8453=ORIENTED_EDGE ( 'NONE', *, *, #15759, .T. ) ;
#8473=VERTEX_POINT ( 'NONE', #10073 ) ;
#8478=ORIENTED_EDGE ( 'NONE', *, *, #9199, .F. ) ;
#8492=CONICAL_SURFACE ( 'NONE', #18380, 0.4863540308881693086, 1.365720138124999927 ) ;
#8547=CARTESIAN_POINT ( 'NONE',  ( 0.1522836969735573143, 0.000000000000000000, 0.000000000000000000 ) ) ;
#8571=ORIENTED_EDGE ( 'NONE', *, *, #22943, .F. ) ;
#8597=ORIENTED_EDGE ( 'NONE', *, *, #26056, .T. ) ;
#8639=CYLINDRICAL_SURFACE ( 'NONE', #26341, 0.4807043897637795493 ) ;
#8641=DIRECTION ( 'NONE',  ( 0.000000000000000000, -1.000000000000000000, 0.000000000000000000 ) ) ;
#8644=EDGE_CURVE ( 'NONE', #15443, #15651, #1893, .T. ) ;
#8656=DIRECTION ( 'NONE',  ( 1.000000000000000000, 0.000000000000000000, 0.000000000000000000 ) ) ;
#8657=DIRECTION ( 'NONE',  ( -0.9790454724845842893, 0.1018208755700880375, -0.1763589297585410332 ) ) ;
#8669=AXIS2_PLACEMENT_3D ( 'NONE', #7795, #10318, #10172 ) ;
#8700=CARTESIAN_POINT ( 'NONE',  ( 0.03937007874015747977, 0.000000000000000000, 0.000000000000000000 ) ) ;
#8727=ORIENTED_EDGE ( 'NONE', *, *, #22521, .T. ) ;
#8736=VECTOR ( 'NONE', #13821, 39.37007874015748143 ) ;
#8761=ORIENTED_EDGE ( 'NONE', *, *, #5290, .T. ) ;
#8775=CARTESIAN_POINT ( 'NONE',  ( 0.4130706566799093316, 0.6693539628600351232, 1.355058665357500095E-17 ) ) ;
#8778=ORIENTED_EDGE ( 'NONE', *, *, #15964, .T. ) ;
#8798=EDGE_LOOP ( 'NONE', ( #228, #18031, #2852, #21172, #8172, #732 ) ) ;
#8802=EDGE_CURVE ( 'NONE', #27102, #4182, #10018, .T. ) ;
#8805=B_SPLINE_CURVE_WITH_KNOTS ( 'NONE', 3,
 ( #7975, #12792, #6580, #17448 ),
 .UNSPECIFIED., .F., .F.,
 ( 4, 4 ),
 ( 1.743059029969430185, 1.744705333033729877 ),
 .UNSPECIFIED. ) ;
#8862=EDGE_CURVE ( 'NONE', #21888, #19645, #4659, .T. ) ;
#8889=CARTESIAN_POINT ( 'NONE',  ( 0.1522836969735572310, -0.4941010236220472751, 6.050992370341708321E-17 ) ) ;
#8890=AXIS2_PLACEMENT_3D ( 'NONE', #18878, #26691, #1658 ) ;
#8896=EDGE_LOOP ( 'NONE', ( #15371, #7415, #19217, #22384 ) ) ;
#8906=LINE ( 'NONE', #19923, #10954 ) ;
#8943=DIRECTION ( 'NONE',  ( -0.9790454724845839563, 0.1018208755700888840, 0.1763589297585419768 ) ) ;
#8992=CARTESIAN_POINT ( 'NONE',  ( 0.1522836969735572310, -0.4941010236220472751, 6.050992370341708321E-17 ) ) ;
#8995=ORIENTED_EDGE ( 'NONE', *, *, #26584, .F. ) ;
#9016=PLANE ( 'NONE',  #19562 ) ;
#9029=ORIENTED_EDGE ( 'NONE', *, *, #24577, .F. ) ;
#9065=AXIS2_PLACEMENT_3D ( 'NONE', #17901, #843, #24554 ) ;
#9098=CARTESIAN_POINT ( 'NONE',  ( 0.1512365935307563025, 0.2842733266362078570, 0.3980489158656032589 ) ) ;
#9133=ADVANCED_FACE ( 'NONE', ( #13282 ), #4179, .T. ) ;
#9140=AXIS2_PLACEMENT_3D ( 'NONE', #27584, #1998, #18949 ) ;
#9141=DIRECTION ( 'NONE',  ( 0.000000000000000000, 1.000000000000000000, 0.000000000000000000 ) ) ;
#9147=CARTESIAN_POINT ( 'NONE',  ( 0.6055690743987126590, 0.2581485381169802973, 0.4471263839182408883 ) ) ;
#9155=DIRECTION ( 'NONE',  ( 0.000000000000000000, 1.000000000000000000, 0.000000000000000000 ) ) ;
#9168=CARTESIAN_POINT ( 'NONE',  ( 0.1490609433615242285, 0.000000000000000000, 0.000000000000000000 ) ) ;
#9187=ORIENTED_EDGE ( 'NONE', *, *, #615, .F. ) ;
#9199=EDGE_CURVE ( 'NONE', #24937, #12967, #3019, .T. ) ;
#9248=ADVANCED_FACE ( 'NONE', ( #14122 ), #23161, .T. ) ;
#9263=AXIS2_PLACEMENT_3D ( 'NONE', #13459, #6985, #4842 ) ;
#9275=ORIENTED_EDGE ( 'NONE', *, *, #6471, .T. ) ;
#9316=LINE ( 'NONE', #2818, #7025 ) ;
#9359=CARTESIAN_POINT ( 'NONE',  ( 0.1517511419330843936, -0.2889986225176974788, -0.3976299462310772248 ) ) ;
#9360=PLANE ( 'NONE',  #13080 ) ;
#9390=ADVANCED_FACE ( 'NONE', ( #13906, #20117 ), #26465, .T. ) ;
#9402=CARTESIAN_POINT ( 'NONE',  ( 0.1512183756281842983, -0.2026803072306157250, -0.4450749096211394362 ) ) ;
#9509=ORIENTED_EDGE ( 'NONE', *, *, #5628, .F. ) ;
#9511=ADVANCED_FACE ( 'NONE', ( #14202 ), #17283, .T. ) ;
#9512=CONICAL_SURFACE ( 'NONE', #26229, 0.4863540308881693086, 1.365720138124999927 ) ;
#9526=ORIENTED_EDGE ( 'NONE', *, *, #5522, .T. ) ;
#9529=ORIENTED_EDGE ( 'NONE', *, *, #18476, .F. ) ;
#9537=DIRECTION ( 'NONE',  ( 0.9790454724845839563, 0.2036417511401769909, -2.493892000000000165E-17 ) ) ;
#9557=LINE ( 'NONE', #7450, #26195 ) ;
#9558=AXIS2_PLACEMENT_3D ( 'NONE', #8700, #6041, #2202 ) ;
#9580=CIRCLE ( 'NONE', #9140, 0.1298643763538141760 ) ;
#9595=CARTESIAN_POINT ( 'NONE',  ( 0.1522836969735573143, -0.4909267390297480382, -0.05591742528025173131 ) ) ;
#9598=AXIS2_PLACEMENT_3D ( 'NONE', #2624, #4488, #17341 ) ;
#9644=EDGE_CURVE ( 'NONE', #19740, #24937, #13153, .T. ) ;
#9653=ORIENTED_EDGE ( 'NONE', *, *, #7386, .F. ) ;
#9656=ORIENTED_EDGE ( 'NONE', *, *, #21085, .F. ) ;
#9660=EDGE_CURVE ( 'NONE', #21106, #16322, #21249, .T. ) ;
#9674=ORIENTED_EDGE ( 'NONE', *, *, #26682, .T. ) ;
#9676=ORIENTED_EDGE ( 'NONE', *, *, #13598, .T. ) ;
#9693=CONICAL_SURFACE ( 'NONE', #2036, 0.4863540308881693086, 1.365720138124999927 ) ;
#9713=AXIS2_PLACEMENT_3D ( 'NONE', #22939, #1455, #25181 ) ;
#9747=FACE_BOUND ( 'NONE', #627, .T. ) ;
#9781=VERTEX_POINT ( 'NONE', #24050 ) ;
#9783=FACE_OUTER_BOUND ( 'NONE', #24580, .T. ) ;
#9789=DIRECTION ( 'NONE',  ( -0.2036417511401762970, -0.9790454724845841783, 0.000000000000000000 ) ) ;
#9810=B_SPLINE_CURVE_WITH_KNOTS ( 'NONE', 3,
 ( #11284, #4919, #13533, #15672 ),
 .UNSPECIFIED., .F., .F.,
 ( 4, 4 ),
 ( 1.726261509291350027, 1.727907812355649941 ),
 .UNSPECIFIED. ) ;
#9818=CARTESIAN_POINT ( 'NONE',  ( 0.000000000000000000, 0.4941010236220472751, 0.000000000000000000 ) ) ;
#9838=CARTESIAN_POINT ( 'NONE',  ( 0.1520645003680120011, 0.1970746732787106437, 0.4530975572029189435 ) ) ;
#9867=EDGE_LOOP ( 'NONE', ( #19076, #4872, #18206, #8995 ) ) ;
#9884=AXIS2_PLACEMENT_3D ( 'NONE', #14045, #20538, #24617 ) ;
#9901=ORIENTED_EDGE ( 'NONE', *, *, #24366, .F. ) ;
#9902=SURFACE_STYLE_USAGE ( .BOTH. , #16403 ) ;
#9910=AXIS2_PLACEMENT_3D ( 'NONE', #915, #5278, #15876 ) ;
#9912=ADVANCED_FACE ( 'NONE', ( #16136 ), #7825, .T. ) ;
#9925=DIRECTION ( 'NONE',  ( -0.2036417511401762970, 0.9790454724845841783, -1.198984999999999849E-16 ) ) ;
#9926=ORIENTED_EDGE ( 'NONE', *, *, #10677, .F. ) ;
#10003=FACE_OUTER_BOUND ( 'NONE', #5027, .T. ) ;
#10018=CIRCLE ( 'NONE', #8669, 0.4941010236220472751 ) ;
#10031=CARTESIAN_POINT ( 'NONE',  ( 0.000000000000000000, -0.4941010236220472751, 6.050992370341708321E-17 ) ) ;
#10042=ADVANCED_FACE ( 'NONE', ( #16273 ), #27224, .T. ) ;
#10051=CARTESIAN_POINT ( 'NONE',  ( 0.6299212598425196763, 0.000000000000000000, 0.000000000000000000 ) ) ;
#10055=CARTESIAN_POINT ( 'NONE',  ( 0.03937007874015747977, 0.000000000000000000, 0.000000000000000000 ) ) ;
#10073=CARTESIAN_POINT ( 'NONE',  ( 0.000000000000000000, 0.000000000000000000, -0.3740157480314960647 ) ) ;
#10117=CARTESIAN_POINT ( 'NONE',  ( 0.1522836969735573143, 0.2938892803217901806, -0.3971963147566898167 ) ) ;
#10136=CARTESIAN_POINT ( 'NONE',  ( 0.1501355178992943018, -0.4826710871606547104, 0.03296692058226987493 ) ) ;
#10172=DIRECTION ( 'NONE',  ( 0.000000000000000000, 1.000000000000000000, 0.000000000000000000 ) ) ;
#10192=EDGE_LOOP ( 'NONE', ( #18703, #16641, #2309, #12533, #10236, #25887 ) ) ;
#10209=DIRECTION ( 'NONE',  ( 0.000000000000000000, -1.000000000000000000, 0.000000000000000000 ) ) ;
#10213=ORIENTED_EDGE ( 'NONE', *, *, #11996, .T. ) ;
#10236=ORIENTED_EDGE ( 'NONE', *, *, #11293, .T. ) ;
#10274=CARTESIAN_POINT ( 'NONE',  ( 0.1490609433494345937, -0.4786070381568061083, 0.009463581268761192544 ) ) ;
#10309=CARTESIAN_POINT ( 'NONE',  ( 0.1522836969735572310, 0.4941010236220472751, 0.000000000000000000 ) ) ;
#10314=( CONVERSION_BASED_UNIT ( 'INCH', #18499 ) LENGTH_UNIT ( ) NAMED_UNIT ( #10500 ) ) ;
#10318=DIRECTION ( 'NONE',  ( 1.000000000000000000, 0.000000000000000000, 0.000000000000000000 ) ) ;
#10333=EDGE_CURVE ( 'NONE', #3752, #2655, #7053, .T. ) ;
#10342=ORIENTED_EDGE ( 'NONE', *, *, #10985, .T. ) ;
#10360=CARTESIAN_POINT ( 'NONE',  ( 0.1490609433615242285, 0.4786070381542913421, 0.000000000000000000 ) ) ;
#10394=LINE ( 'NONE', #16617, #20684 ) ;
#10395=DIRECTION ( 'NONE',  ( 0.000000000000000000, -1.000000000000000000, 0.000000000000000000 ) ) ;
#10405=ORIENTED_EDGE ( 'NONE', *, *, #2278, .F. ) ;
#10425=AXIS2_PLACEMENT_3D ( 'NONE', #25812, #23965, #4340 ) ;
#10431=ORIENTED_EDGE ( 'NONE', *, *, #4721, .F. ) ;
#10459=CARTESIAN_POINT ( 'NONE',  ( 0.1638952246732497953, -0.5499255957412874096, 6.734645669291338471E-17 ) ) ;
#10464=CARTESIAN_POINT ( 'NONE',  ( 0.6055690743987126590, -0.2581485381169807414, -0.4471263839182408883 ) ) ;
#10482=FACE_OUTER_BOUND ( 'NONE', #23618, .T. ) ;
#10500=DIMENSIONAL_EXPONENTS ( 1.000000000000000000, 0.000000000000000000, 0.000000000000000000, 0.000000000000000000, 0.000000000000000000, 0.000000000000000000, 0.000000000000000000 ) ;
#10516=DIRECTION ( 'NONE',  ( 1.000000000000000000, 0.000000000000000000, 0.000000000000000000 ) ) ;
#10518=ADVANCED_FACE ( 'NONE', ( #4213 ), #10553, .F. ) ;
#10542=ORIENTED_EDGE ( 'NONE', *, *, #20406, .F. ) ;
#10553=CYLINDRICAL_SURFACE ( 'NONE', #1908, 0.3346456692913385988 ) ;
#10559=DIRECTION ( 'NONE',  ( 1.000000000000000000, 0.000000000000000000, 0.000000000000000000 ) ) ;
#10583=ORIENTED_EDGE ( 'NONE', *, *, #16080, .F. ) ;
#10603=ORIENTED_EDGE ( 'NONE', *, *, #18237, .F. ) ;
#10604=DIRECTION ( 'NONE',  ( -0.9790454724845842893, -0.1018208755700880375, -0.1763589297585410332 ) ) ;
#10616=EDGE_CURVE ( 'NONE', #25542, #12210, #11742, .T. ) ;
#10645=CIRCLE ( 'NONE', #3895, 0.03937007874015744507 ) ;
#10677=EDGE_CURVE ( 'NONE', #11062, #24440, #19952, .T. ) ;
#10696=CARTESIAN_POINT ( 'NONE',  ( 0.6055690743987126590, -0.2581485381169807414, -0.4471263839182408883 ) ) ;
#10704=ORIENTED_EDGE ( 'NONE', *, *, #2195, .T. ) ;
#10714=AXIS2_PLACEMENT_3D ( 'NONE', #5136, #22240, #781 ) ;
#10720=CARTESIAN_POINT ( 'NONE',  ( 0.1490609433615242285, -0.2393035190771456711, -0.4144858534716441278 ) ) ;
#10725=CARTESIAN_POINT ( 'NONE',  ( 0.1520645003680120011, -0.4909313315697558799, -0.05587710509957795335 ) ) ;
#10726=CARTESIAN_POINT ( 'NONE',  ( 0.1512365701434773002, -0.2842731118987109618, 0.3980489349105370556 ) ) ;
#10751=ADVANCED_FACE ( 'NONE', ( #20422 ), #13172, .T. ) ;
#10752=ORIENTED_EDGE ( 'NONE', *, *, #5465, .T. ) ;
#10794=EDGE_LOOP ( 'NONE', ( #3437, #5979, #6990 ) ) ;
#10797=PLANE ( 'NONE',  #11815 ) ;
#10821=CARTESIAN_POINT ( 'NONE',  ( 0.1516263115863346334, 0.1971492568089275588, 0.4530651079966787620 ) ) ;
#10826=DIRECTION ( 'NONE',  ( -0.9790454724845839563, 0.2036417511401769909, 0.000000000000000000 ) ) ;
#10856=ORIENTED_EDGE ( 'NONE', *, *, #14054, .F. ) ;
#10859=CARTESIAN_POINT ( 'NONE',  ( 0.1522836969815822838, -0.2938892803218252081, 0.3971963147669425598 ) ) ;
#10897=CIRCLE ( 'NONE', #21267, 0.09143349766193348271 ) ;
#10901=DIRECTION ( 'NONE',  ( 1.000000000000000000, 0.000000000000000000, 0.000000000000000000 ) ) ;
#10918=DIRECTION ( 'NONE',  ( -0.9790454724845840673, 0.1018208755700876073, -0.1763589297585415050 ) ) ;
#10923=LINE ( 'NONE', #17681, #15296 ) ;
#10941=DIRECTION ( 'NONE',  ( -0.9790454724845842893, 0.1018208755700880375, 0.1763589297585410332 ) ) ;
#10954=VECTOR ( 'NONE', #714, 39.37007874015748143 ) ;
#10967=LINE ( 'NONE', #19593, #8182 ) ;
#10985=EDGE_CURVE ( 'NONE', #18210, #19765, #23611, .T. ) ;
#11023=VERTEX_POINT ( 'NONE', #12051 ) ;
#11025=FACE_OUTER_BOUND ( 'NONE', #27422, .T. ) ;
#11054=VERTEX_POINT ( 'NONE', #907 ) ;
#11062=VERTEX_POINT ( 'NONE', #18530 ) ;
#11064=DIRECTION ( 'NONE',  ( -0.9790454724845839563, -0.1018208755700890228, -0.1763589297585420324 ) ) ;
#11067=AXIS2_PLACEMENT_3D ( 'NONE', #27241, #11836, #7607 ) ;
#11073=ADVANCED_FACE ( 'NONE', ( #16161 ), #5541, .T. ) ;
#11108=ORIENTED_EDGE ( 'NONE', *, *, #17282, .T. ) ;
#11135=CARTESIAN_POINT ( 'NONE',  ( 0.1504231045792248644, -0.2747315525089227273, 0.3999795527262415273 ) ) ;
#11137=CARTESIAN_POINT ( 'NONE',  ( 0.5869493968219645641, 0.2133897621573074832, 0.3696019098714952711 ) ) ;
#11148=CARTESIAN_POINT ( 'NONE',  ( 0.5981657849660177995, 0.000000000000000000, 0.000000000000000000 ) ) ;
#11165=DIRECTION ( 'NONE',  ( -0.2036417511401761582, 0.4895227362422917006, -0.8478782506317886769 ) ) ;
#11188=CARTESIAN_POINT ( 'NONE',  ( 0.1516263115863346334, 0.2937912646890004087, -0.3972688187320929099 ) ) ;
#11202=AXIS2_PLACEMENT_3D ( 'NONE', #2404, #4403, #6665 ) ;
#11210=DIRECTION ( 'NONE',  ( -1.000000000000000000, 0.000000000000000000, 0.000000000000000000 ) ) ;
#11224=ADVANCED_FACE ( 'NONE', ( #12886 ), #14139, .F. ) ;
#11225=VECTOR ( 'NONE', #4833, 39.37007874015748143 ) ;
#11246=CIRCLE ( 'NONE', #24774, 0.09143349766193348271 ) ;
#11250=DIRECTION ( 'NONE',  ( -0.2036417511401760472, 0.9790454724845840673, -1.198985000000000095E-16 ) ) ;
#11284=CARTESIAN_POINT ( 'NONE',  ( 0.1516263115863346334, -0.4909405214979283838, 0.05579628926458630317 ) ) ;
#11293=EDGE_CURVE ( 'NONE', #4526, #9781, #7822, .T. ) ;
#11309=CARTESIAN_POINT ( 'NONE',  ( 0.1522836969735573143, 0.2938892803217905692, 0.3971963147566898167 ) ) ;
#11331=CARTESIAN_POINT ( 'NONE',  ( 0.03937007874015747977, 0.000000000000000000, 0.000000000000000000 ) ) ;
#11360=CARTESIAN_POINT ( 'NONE',  ( 0.1516263115863346334, -0.1971492568089271424, 0.4530651079966787620 ) ) ;
#11406=AXIS2_PLACEMENT_3D ( 'NONE', #20481, #7633, #20762 ) ;
#11415=DIRECTION ( 'NONE',  ( -0.2036417511401758251, -0.4895227362422921447, -0.8478782506317885659 ) ) ;
#11421=CARTESIAN_POINT ( 'NONE',  ( 0.5869493968219645641, 0.4267795243146149664, 0.000000000000000000 ) ) ;
#11430=CIRCLE ( 'NONE', #27233, 0.09143349766193348271 ) ;
#11432=CARTESIAN_POINT ( 'NONE',  ( 0.3905379133858267737, 0.5610236220472440971, 0.000000000000000000 ) ) ;
#11439=CARTESIAN_POINT ( 'NONE',  ( 0.1518453844022533417, 0.4909359254662000183, -0.05583672883938756160 ) ) ;
#11448=VECTOR ( 'NONE', #20797, 39.37007874015748854 ) ;
#11452=VERTEX_POINT ( 'NONE', #23450 ) ;
#11456=DIRECTION ( 'NONE',  ( 0.000000000000000000, 1.000000000000000000, 0.000000000000000000 ) ) ;
#11460=ORIENTED_EDGE ( 'NONE', *, *, #18237, .T. ) ;
#11497=CARTESIAN_POINT ( 'NONE',  ( 0.1512834625131516675, -0.2841833823079704668, -0.3983296490053409022 ) ) ;
#11498=FACE_OUTER_BOUND ( 'NONE', #1760, .T. ) ;
#11499=CARTESIAN_POINT ( 'NONE',  ( 0.1490609433537086470, 0.2308937649799950309, 0.4193412272900834958 ) ) ;
#11525=ORIENTED_EDGE ( 'NONE', *, *, #21299, .F. ) ;
#11532=CONICAL_SURFACE ( 'NONE', #15174, 0.4526932812344527379, 0.1178097243749990780 ) ;
#11540=CARTESIAN_POINT ( 'NONE',  ( 0.5981657849660177995, -0.4807043897637795493, 5.886929133858268250E-17 ) ) ;
#11553=LINE ( 'NONE', #3203, #8736 ) ;
#11567=CARTESIAN_POINT ( 'NONE',  ( 0.1522836969735573143, 0.4909267390297480382, -0.05591742528025173131 ) ) ;
#11580=CARTESIAN_POINT ( 'NONE',  ( 0.5869493968219645641, -0.2133897621573078718, -0.3696019098714952711 ) ) ;
#11591=CARTESIAN_POINT ( 'NONE',  ( 0.1525037638700916243, -0.2314035372547590674, -0.4381595109572583580 ) ) ;
#11593=DIRECTION ( 'NONE',  ( 1.000000000000000000, 0.000000000000000000, 0.000000000000000000 ) ) ;
#11602=ORIENTED_EDGE ( 'NONE', *, *, #12114, .F. ) ;
#11614=CARTESIAN_POINT ( 'NONE',  ( 0.1522836969735572310, -0.4941010236220472751, 6.050992370341708321E-17 ) ) ;
#11638=DIRECTION ( 'NONE',  ( 1.000000000000000000, 0.000000000000000000, 0.000000000000000000 ) ) ;
#11642=CONICAL_SURFACE ( 'NONE', #8057, 0.1106489370078740098, 0.08726646250000029414 ) ;
#11643=VERTEX_POINT ( 'NONE', #21863 ) ;
#11666=ORIENTED_EDGE ( 'NONE', *, *, #15433, .T. ) ;
#11668=ORIENTED_EDGE ( 'NONE', *, *, #8644, .F. ) ;
#11683=CARTESIAN_POINT ( 'NONE',  ( 0.1517511419331057931, 0.1998583234825911659, -0.4490951218747354923 ) ) ;
#11697=CARTESIAN_POINT ( 'NONE',  ( 0.1506723201675407575, 0.000000000000000000, 0.000000000000000000 ) ) ;
#11723=CARTESIAN_POINT ( 'NONE',  ( 0.1516263115863346334, 0.2937912646890007973, 0.3972688187320929099 ) ) ;
#11742=B_SPLINE_CURVE_WITH_KNOTS ( 'NONE', 3,
 ( #20004, #525, #26628, #26091, #24507, #6752, #17475, #4607 ),
 .UNSPECIFIED., .F., .F.,
 ( 4, 2, 2, 4 ),
 ( 0.000000000000000000, 0.2500000000000002776, 0.5000000000000005551, 1.000000000000000000 ),
 .UNSPECIFIED. ) ;
#11747=CARTESIAN_POINT ( 'NONE',  ( 0.1522836969735573143, -0.4909267390297480382, 0.05591742528025181458 ) ) ;
#11761=DIRECTION ( 'NONE',  ( -0.9790454724845842893, 0.1018208755700880375, 0.1763589297585410332 ) ) ;
#11762=ORIENTED_EDGE ( 'NONE', *, *, #2969, .T. ) ;
#11764=( LENGTH_UNIT ( ) NAMED_UNIT ( * ) SI_UNIT ( $, .METRE. ) ) ;
#11776=CARTESIAN_POINT ( 'NONE',  ( 0.1490609433576163545, -0.2393035190829114200, 0.4144858534816307505 ) ) ;
#11812=DIRECTION ( 'NONE',  ( 0.000000000000000000, -1.224646707287115868E-16, -1.000000000000000000 ) ) ;
#11815=AXIS2_PLACEMENT_3D ( 'NONE', #19415, #8943, #13181 ) ;
#11830=DIRECTION ( 'NONE',  ( 0.000000000000000000, 1.000000000000000000, 0.000000000000000000 ) ) ;
#11836=DIRECTION ( 'NONE',  ( 0.000000000000000000, 1.000000000000000000, -1.224646799147353207E-16 ) ) ;
#11911=CARTESIAN_POINT ( 'NONE',  ( 0.3905379133858267737, 0.5610236220472440971, 0.000000000000000000 ) ) ;
#11921=CARTESIAN_POINT ( 'NONE',  ( 0.1490609433494345937, -0.2474992208661806470, -0.4097540628404507945 ) ) ;
#11996=EDGE_CURVE ( 'NONE', #1231, #19596, #15812, .T. ) ;
#11997=CARTESIAN_POINT ( 'NONE',  ( 0.1490609433494345937, 0.4786070381568061083, -0.009463581267948129386 ) ) ;
#12006=DIRECTION ( 'NONE',  ( 0.000000000000000000, 1.000000000000000000, 0.000000000000000000 ) ) ;
#12009=VECTOR ( 'NONE', #23077, 39.37007874015748854 ) ;
#12024=B_SPLINE_CURVE_WITH_KNOTS ( 'NONE', 3,
 ( #6056, #1004, #25389, #12540, #5911, #20487, #1146, #9595 ),
 .UNSPECIFIED., .F., .F.,
 ( 4, 2, 2, 4 ),
 ( 0.000000000000000000, 0.2499999999999998890, 0.4999999999999997780, 1.000000000000000000 ),
 .UNSPECIFIED. ) ;
#12025=FACE_OUTER_BOUND ( 'NONE', #18987, .T. ) ;
#12030=EDGE_CURVE ( 'NONE', #26980, #24440, #17252, .T. ) ;
#12039=ORIENTED_EDGE ( 'NONE', *, *, #3964, .F. ) ;
#12051=CARTESIAN_POINT ( 'NONE',  ( 0.1490609433615242285, -0.2393035190771456711, -0.4144858534716441278 ) ) ;
#12114=EDGE_CURVE ( 'NONE', #15651, #25542, #9557, .T. ) ;
#12133=ORIENTED_EDGE ( 'NONE', *, *, #4241, .F. ) ;
#12134=CARTESIAN_POINT ( 'NONE',  ( 0.5869493968219645641, -0.2133897621573078718, -0.3696019098714952711 ) ) ;
#12136=UNCERTAINTY_MEASURE_WITH_UNIT (LENGTH_MEASURE( 1.000000000000000082E-05 ), #10314, 'distance_accuracy_value', 'NONE') ;
#12141=COLOUR_RGB ( '', 0.66274510, 0.83137255, 0.94901961) ;
#12178=EDGE_CURVE ( 'NONE', #16783, #9781, #5910, .T. ) ;
#12190=CIRCLE ( 'NONE', #21683, 0.03937007874015744507 ) ;
#12205=VERTEX_POINT ( 'NONE', #6598 ) ;
#12210=VERTEX_POINT ( 'NONE', #23568 ) ;
#12213=ORIENTED_EDGE ( 'NONE', *, *, #8260, .F. ) ;
#12239=CARTESIAN_POINT ( 'NONE',  ( 0.1520645003680120011, 0.2938566582910456804, -0.3972204521033417812 ) ) ;
#12276=EDGE_LOOP ( 'NONE', ( #24684, #17074, #15910, #6676 ) ) ;
#12297=VERTEX_POINT ( 'NONE', #4336 ) ;
#12298=DIRECTION ( 'NONE',  ( 0.000000000000000000, 1.000000000000000000, 0.000000000000000000 ) ) ;
#12310=EDGE_CURVE ( 'NONE', #11643, #19740, #10967, .T. ) ;
#12344=CARTESIAN_POINT ( 'NONE',  ( 0.4130706566799093316, -0.3346769814300175616, 0.5796775359605756961 ) ) ;
#12351=EDGE_CURVE ( 'NONE', #11643, #22824, #3187, .T. ) ;
#12374=LINE ( 'NONE', #25086, #2783 ) ;
#12380=CARTESIAN_POINT ( 'NONE',  ( 0.1518453843511950729, 0.2938239883646059369, -0.3972446186700991921 ) ) ;
#12393=CARTESIAN_POINT ( 'NONE',  ( 0.6055690743987126590, 0.2581485381169799642, -0.4471263839182408883 ) ) ;
#12403=CARTESIAN_POINT ( 'NONE',  ( 0.5905511811023621549, 0.000000000000000000, 0.000000000000000000 ) ) ;
#12416=ORIENTED_EDGE ( 'NONE', *, *, #15042, .T. ) ;
#12438=VERTEX_POINT ( 'NONE', #22674 ) ;
#12443=CARTESIAN_POINT ( 'NONE',  ( 0.5905511811023621549, 0.000000000000000000, -0.3740157480314960647 ) ) ;
#12451=AXIS2_PLACEMENT_3D ( 'NONE', #11432, #6662, #20052 ) ;
#12483=ORIENTED_EDGE ( 'NONE', *, *, #18476, .T. ) ;
#12492=EDGE_CURVE ( 'NONE', #21046, #23841, #26479, .T. ) ;
#12494=UNCERTAINTY_MEASURE_WITH_UNIT (LENGTH_MEASURE( 1.000000000000000082E-05 ), #904, 'distance_accuracy_value', 'NONE') ;
#12503=ORIENTED_EDGE ( 'NONE', *, *, #20952, .F. ) ;
#12524=AXIS2_PLACEMENT_3D ( 'NONE', #2291, #10918, #4557 ) ;
#12533=ORIENTED_EDGE ( 'NONE', *, *, #21382, .F. ) ;
#12540=CARTESIAN_POINT ( 'NONE',  ( 0.1493967478962656692, -0.4798749592428788180, -0.01883130896440190702 ) ) ;
#12557=ORIENTED_EDGE ( 'NONE', *, *, #19567, .F. ) ;
#12558=ORIENTED_EDGE ( 'NONE', *, *, #25273, .T. ) ;
#12561=AXIS2_PLACEMENT_3D ( 'NONE', #7214, #15832, #24308 ) ;
#12566=FACE_OUTER_BOUND ( 'NONE', #16555, .T. ) ;
#12569=TOROIDAL_SURFACE ( 'NONE', #8062, 0.3740157480314960647, 0.03937007874015747977 ) ;
#12610=CONICAL_SURFACE ( 'NONE', #5382, 0.1106489370078740930, 0.08726646250000029414 ) ;
#12629=CARTESIAN_POINT ( 'NONE',  ( 0.1504127680534947942, 0.4837205684772488690, 0.03783905811611818631 ) ) ;
#12669=CARTESIAN_POINT ( 'NONE',  ( 0.5869493968219645641, 0.2133897621573074832, 0.3696019098714952711 ) ) ;
#12673=ADVANCED_FACE ( 'NONE', ( #4570 ), #10797, .T. ) ;
#12691=VERTEX_POINT ( 'NONE', #15188 ) ;
#12710=DIRECTION ( 'NONE',  ( -0.2036417511401763802, 0.4895227362422922557, 0.8478782506317883438 ) ) ;
#12742=AXIS2_PLACEMENT_3D ( 'NONE', #5003, #13624, #20266 ) ;
#12769=DIRECTION ( 'NONE',  ( -0.9790454724845842893, 0.2036417511401760472, 0.000000000000000000 ) ) ;
#12779=AXIS2_PLACEMENT_3D ( 'NONE', #6331, #25256, #14963 ) ;
#12784=ORIENTED_EDGE ( 'NONE', *, *, #21668, .T. ) ;
#12792=CARTESIAN_POINT ( 'NONE',  ( 0.1518453844022533417, -0.2938239883722331136, -0.3972446186644590371 ) ) ;
#12798=CARTESIAN_POINT ( 'NONE',  ( 0.5981657849660177995, 0.000000000000000000, 0.000000000000000000 ) ) ;
#12833=AXIS2_PLACEMENT_3D ( 'NONE', #22936, #14469, #23078 ) ;
#12844=ORIENTED_EDGE ( 'NONE', *, *, #2597, .T. ) ;
#12865=AXIS2_PLACEMENT_3D ( 'NONE', #19631, #17496, #6773 ) ;
#12886=FACE_OUTER_BOUND ( 'NONE', #15656, .T. ) ;
#12892=AXIS2_PLACEMENT_3D ( 'NONE', #8547, #17433, #21818 ) ;
#12947=VERTEX_POINT ( 'NONE', #24426 ) ;
#12967=VERTEX_POINT ( 'NONE', #2800 ) ;
#12982=ORIENTED_EDGE ( 'NONE', *, *, #24353, .T. ) ;
#12999=DIRECTION ( 'NONE',  ( 0.000000000000000000, 1.000000000000000000, 0.000000000000000000 ) ) ;
#13035=FACE_OUTER_BOUND ( 'NONE', #22546, .T. ) ;
#13037=B_SPLINE_CURVE_WITH_KNOTS ( 'NONE', 3,
 ( #16742, #4308, #15219, #25504 ),
 .UNSPECIFIED., .F., .F.,
 ( 4, 4 ),
 ( 1.006307675027575899, 1.007953978091874037 ),
 .UNSPECIFIED. ) ;
#13065=ORIENTED_EDGE ( 'NONE', *, *, #14772, .T. ) ;
#13080=AXIS2_PLACEMENT_3D ( 'NONE', #16305, #27185, #20395 ) ;
#13098=VERTEX_POINT ( 'NONE', #19586 ) ;
#13114=EDGE_CURVE ( 'NONE', #19596, #24341, #23584, .T. ) ;
#13144=DIRECTION ( 'NONE',  ( 1.000000000000000000, 0.000000000000000000, 0.000000000000000000 ) ) ;
#13153=B_SPLINE_CURVE_WITH_KNOTS ( 'NONE', 3,
 ( #10360, #27193, #4153, #18684, #23386, #12629, #7839, #27327 ),
 .UNSPECIFIED., .F., .F.,
 ( 4, 2, 2, 4 ),
 ( 0.000000000000000000, 0.2499999999999997780, 0.4999999999999995559, 1.000000000000000000 ),
 .UNSPECIFIED. ) ;
#13159=CARTESIAN_POINT ( 'NONE',  ( 0.1506723201675407575, 0.000000000000000000, 0.000000000000000000 ) ) ;
#13170=FACE_OUTER_BOUND ( 'NONE', #7210, .T. ) ;
#13172=CONICAL_SURFACE ( 'NONE', #4195, 0.4537419570391968415, 1.365720138124999927 ) ;
#13181=DIRECTION ( 'NONE',  ( 0.1034422368825631960, 0.9946354626840587798, 0.000000000000000000 ) ) ;
#13250=CARTESIAN_POINT ( 'NONE',  ( 0.6055690743987126590, 0.5162970762339605946, 0.000000000000000000 ) ) ;
#13282=FACE_OUTER_BOUND ( 'NONE', #7993, .T. ) ;
#13293=ADVANCED_FACE ( 'NONE', ( #22385 ), #21349, .T. ) ;
#13303=DIRECTION ( 'NONE',  ( -0.9575713608335526539, 0.1440981340193014382, 0.2495852893972990150 ) ) ;
#13341=CARTESIAN_POINT ( 'NONE',  ( 0.1516263115863346334, 0.1971492568089271424, -0.4530651079966795947 ) ) ;
#13347=DIRECTION ( 'NONE',  ( 0.000000000000000000, 1.000000000000000000, 0.000000000000000000 ) ) ;
#13369=CONICAL_SURFACE ( 'NONE', #2964, 0.4526932812344527379, 0.1178097243749990780 ) ;
#13414=AXIS2_PLACEMENT_3D ( 'NONE', #17411, #8656, #17279 ) ;
#13427=CARTESIAN_POINT ( 'NONE',  ( 0.1516263115863346334, -0.2937912646890007973, -0.3972688187320929099 ) ) ;
#13432=LINE ( 'NONE', #2558, #25233 ) ;
#13459=CARTESIAN_POINT ( 'NONE',  ( 0.07614184848677874040, 0.000000000000000000, 0.000000000000000000 ) ) ;
#13478=CARTESIAN_POINT ( 'NONE',  ( 0.1504366439317611215, 0.2749075979901894895, 0.3999374451793131779 ) ) ;
#13492=EDGE_CURVE ( 'NONE', #17206, #17635, #9580, .T. ) ;
#13497=CARTESIAN_POINT ( 'NONE',  ( 0.1755067523729419432, -0.6057501678605275997, 7.418299212598425247E-17 ) ) ;
#13506=DIRECTION ( 'NONE',  ( 0.000000000000000000, -1.000000000000000000, 0.000000000000000000 ) ) ;
#13529=CARTESIAN_POINT ( 'NONE',  ( 0.5925575908939920700, -0.2268709785195988371, -0.3929520615588121824 ) ) ;
#13533=CARTESIAN_POINT ( 'NONE',  ( 0.1520645003235147619, -0.4909313315706889669, 0.05587710509139291737 ) ) ;
#13534=ORIENTED_EDGE ( 'NONE', *, *, #4130, .T. ) ;
#13561=B_SPLINE_CURVE_WITH_KNOTS ( 'NONE', 3,
 ( #21836, #9098, #13478, #2736, #7131, #26610 ),
 .UNSPECIFIED., .F., .F.,
 ( 4, 2, 4 ),
 ( 8.213553798819532080E-14, 0.0007294428068852555104, 0.001458885613688375334 ),
 .UNSPECIFIED. ) ;
#13580=DIRECTION ( 'NONE',  ( 0.000000000000000000, 0.000000000000000000, -1.000000000000000000 ) ) ;
#13596=DIRECTION ( 'NONE',  ( 1.000000000000000000, 0.000000000000000000, 0.000000000000000000 ) ) ;
#13598=EDGE_CURVE ( 'NONE', #15443, #8047, #8906, .T. ) ;
#13613=CARTESIAN_POINT ( 'NONE',  ( 0.1490609433615242285, -0.2393035190771456711, -0.4144858534716441278 ) ) ;
#13624=DIRECTION ( 'NONE',  ( 1.000000000000000000, 0.000000000000000000, 0.000000000000000000 ) ) ;
#13632=AXIS2_PLACEMENT_3D ( 'NONE', #25046, #22368, #9925 ) ;
#13687=CARTESIAN_POINT ( 'NONE',  ( 0.1517511419331485645, 0.4888569460006513268, -0.05146517564403369632 ) ) ;
#13694=CLOSED_SHELL ( 'NONE', ( #21748, #26920, #17656, #6097, #25240, #2518, #26204, #9912, #19879, #3228, #356, #16343, #2264, #16454, #9390, #14206, #27717, #10518, #4776, #17632, #19889, #6243, #150, #8076, #15587, #11224, #22065, #18707, #17323, #2912, #19752, #19977, #22810, #14325, #27198, #10751, #10042, #9248, #13293, #12673, #9511, #13980, #21856, #9133, #16924, #17450, #11073, #22973, #6040, #1752, #22586, #23906, #17333, #2942 ) ) ;
#13719=DIRECTION ( 'NONE',  ( 0.000000000000000000, 1.000000000000000000, 0.000000000000000000 ) ) ;
#13720=ORIENTED_EDGE ( 'NONE', *, *, #19567, .T. ) ;
#13737=VERTEX_POINT ( 'NONE', #11580 ) ;
#13740=DIRECTION ( 'NONE',  ( -0.2036417511401759084, -0.4895227362422917006, -0.8478782506317888989 ) ) ;
#13743=FACE_OUTER_BOUND ( 'NONE', #3348, .T. ) ;
#13763=FACE_OUTER_BOUND ( 'NONE', #17270, .T. ) ;
#13789=CIRCLE ( 'NONE', #8382, 0.3740157480314960647 ) ;
#13794=FACE_OUTER_BOUND ( 'NONE', #9867, .T. ) ;
#13810=CARTESIAN_POINT ( 'NONE',  ( 0.1490609433494345659, 0.2311078172902765182, -0.4192176441073949267 ) ) ;
#13821=DIRECTION ( 'NONE',  ( 1.000000000000000000, 0.000000000000000000, 0.000000000000000000 ) ) ;
#13824=DIRECTION ( 'NONE',  ( 0.000000000000000000, 1.000000000000000000, 0.000000000000000000 ) ) ;
#13838=EDGE_CURVE ( 'NONE', #7492, #2655, #26310, .T. ) ;
#13842=EDGE_CURVE ( 'NONE', #22807, #21046, #21368, .T. ) ;
#13848=CARTESIAN_POINT ( 'NONE',  ( 0.1518453844022533417, 0.2938239883722331136, 0.3972446186644590371 ) ) ;
#13859=CYLINDRICAL_SURFACE ( 'NONE', #25274, 0.4807043897637795493 ) ;
#13869=VECTOR ( 'NONE', #22106, 39.37007874015748143 ) ;
#13906=FACE_BOUND ( 'NONE', #25968, .T. ) ;
#13909=DIRECTION ( 'NONE',  ( 1.000000000000000000, 0.000000000000000000, 0.000000000000000000 ) ) ;
#13980=ADVANCED_FACE ( 'NONE', ( #12566 ), #21330, .T. ) ;
#14003=DIRECTION ( 'NONE',  ( 0.000000000000000000, 0.000000000000000000, -1.000000000000000000 ) ) ;
#14023=PLANE ( 'NONE',  #14156 ) ;
#14045=CARTESIAN_POINT ( 'NONE',  ( 0.5981657849660177995, 0.000000000000000000, 0.000000000000000000 ) ) ;
#14054=EDGE_CURVE ( 'NONE', #7492, #15470, #23788, .T. ) ;
#14060=ORIENTED_EDGE ( 'NONE', *, *, #26584, .T. ) ;
#14101=DIRECTION ( 'NONE',  ( 0.9930684569549264040, -0.1175373974578370340, 0.000000000000000000 ) ) ;
#14108=EDGE_LOOP ( 'NONE', ( #24174, #14547, #18531, #23188, #463 ) ) ;
#14115=ORIENTED_EDGE ( 'NONE', *, *, #17282, .F. ) ;
#14122=FACE_OUTER_BOUND ( 'NONE', #12276, .T. ) ;
#14139=CONICAL_SURFACE ( 'NONE', #24049, 0.4863540308881693086, 1.365720138124999927 ) ;
#14149=DIRECTION ( 'NONE',  ( 1.000000000000000000, 0.000000000000000000, 0.000000000000000000 ) ) ;
#14156=AXIS2_PLACEMENT_3D ( 'NONE', #748, #10826, #22496 ) ;
#14181=VECTOR ( 'NONE', #23499, 39.37007874015748854 ) ;
#14188=ORIENTED_EDGE ( 'NONE', *, *, #9199, .T. ) ;
#14198=FACE_OUTER_BOUND ( 'NONE', #17479, .T. ) ;
#14202=FACE_OUTER_BOUND ( 'NONE', #21453, .T. ) ;
#14206=ADVANCED_FACE ( 'NONE', ( #3048 ), #19999, .T. ) ;
#14262=CARTESIAN_POINT ( 'NONE',  ( 0.1490609433615242285, -0.4786070381542913421, 5.861244094488189820E-17 ) ) ;
#14315=ORIENTED_EDGE ( 'NONE', *, *, #5465, .F. ) ;
#14325=ADVANCED_FACE ( 'NONE', ( #18302 ), #14637, .T. ) ;
#14349=AXIS2_PLACEMENT_3D ( 'NONE', #22662, #27047, #18543 ) ;
#14374=CIRCLE ( 'NONE', #1707, 0.4807043897637795493 ) ;
#14375=AXIS2_PLACEMENT_3D ( 'NONE', #18803, #27728, #19090 ) ;
#14380=PLANE ( 'NONE',  #873 ) ;
#14430=( BOUNDED_CURVE ( )  B_SPLINE_CURVE ( 3, ( #4814, #11591, #18055, #13427 ),
 .UNSPECIFIED., .F., .T. ) 
 B_SPLINE_CURVE_WITH_KNOTS ( ( 4, 4 ),
 ( 3.028426401679942259, 3.254758905499644417 ),
 .UNSPECIFIED. ) 
 CURVE ( )  GEOMETRIC_REPRESENTATION_ITEM ( )  RATIONAL_B_SPLINE_CURVE ( ( 1.000000000000000000, 0.9957356870045847019, 0.9957356870045847019, 1.000000000000000000 ) ) 
 REPRESENTATION_ITEM ( '' )  ) ;
#14434=ORIENTED_EDGE ( 'NONE', *, *, #19173, .F. ) ;
#14462=ORIENTED_EDGE ( 'NONE', *, *, #10333, .T. ) ;
#14469=DIRECTION ( 'NONE',  ( -1.000000000000000000, 0.000000000000000000, 0.000000000000000000 ) ) ;
#14481=CARTESIAN_POINT ( 'NONE',  ( 0.1512365701434774945, 0.2025839336325081785, 0.4452122039724091263 ) ) ;
#14498=ORIENTED_EDGE ( 'NONE', *, *, #15042, .F. ) ;
#14518=B_SPLINE_CURVE_WITH_KNOTS ( 'NONE', 3,
 ( #23281, #3909, #20586, #1241 ),
 .UNSPECIFIED., .F., .F.,
 ( 4, 4 ),
 ( 1.006307675027575899, 1.007953978091874037 ),
 .UNSPECIFIED. ) ;
#14538=DIRECTION ( 'NONE',  ( -0.2036417511401760472, -0.9790454724845840673, 0.000000000000000000 ) ) ;
#14544=FACE_OUTER_BOUND ( 'NONE', #5982, .T. ) ;
#14547=ORIENTED_EDGE ( 'NONE', *, *, #2115, .T. ) ;
#14571=EDGE_LOOP ( 'NONE', ( #18166, #10213, #14640, #24438, #2254 ) ) ;
#14573=CARTESIAN_POINT ( 'NONE',  ( 0.1490609433576163545, -0.2393035190829114200, 0.4144858534816307505 ) ) ;
#14585=EDGE_CURVE ( 'NONE', #17275, #16783, #25168, .T. ) ;
#14598=VERTEX_POINT ( 'NONE', #18518 ) ;
#14616=VECTOR ( 'NONE', #23322, 39.37007874015748143 ) ;
#14637=CONICAL_SURFACE ( 'NONE', #2413, 0.4526932812344527379, 0.1178097243749990780 ) ;
#14640=ORIENTED_EDGE ( 'NONE', *, *, #13114, .T. ) ;
#14645=AXIS2_PLACEMENT_3D ( 'NONE', #17262, #10901, #206 ) ;
#14664=ORIENTED_EDGE ( 'NONE', *, *, #10616, .T. ) ;
#14715=CONICAL_SURFACE ( 'NONE', #7925, 0.1106489370078739681, 0.08726646250000029414 ) ;
#14717=LINE ( 'NONE', #12134, #14616 ) ;
#14767=DIRECTION ( 'NONE',  ( -1.000000000000000000, 0.000000000000000000, 0.000000000000000000 ) ) ;
#14772=EDGE_CURVE ( 'NONE', #7184, #18835, #4268, .T. ) ;
#14775=CARTESIAN_POINT ( 'NONE',  ( 0.2019525613798653363, -0.3664466487725785981, -0.6347042139374527991 ) ) ;
#14781=VECTOR ( 'NONE', #21277, 39.37007874015748854 ) ;
#14823=B_SPLINE_CURVE_WITH_KNOTS ( 'NONE', 3,
 ( #11723, #13848, #17795, #11309 ),
 .UNSPECIFIED., .F., .F.,
 ( 4, 4 ),
 ( 1.743059029969430185, 1.744705333033729877 ),
 .UNSPECIFIED. ) ;
#14849=DIRECTION ( 'NONE',  ( 0.000000000000000000, -0.8660254037844384856, 0.5000000000000003331 ) ) ;
#14859=EDGE_CURVE ( 'NONE', #23305, #13098, #20125, .T. ) ;
#14917=B_SPLINE_CURVE_WITH_KNOTS ( 'NONE', 3,
 ( #10117, #12239, #12380, #4053 ),
 .UNSPECIFIED., .F., .F.,
 ( 4, 4 ),
 ( 1.006307675027575899, 1.007953978091874037 ),
 .UNSPECIFIED. ) ;
#14944=FACE_OUTER_BOUND ( 'NONE', #8798, .T. ) ;
#14963=DIRECTION ( 'NONE',  ( 0.000000000000000000, 1.000000000000000000, 0.000000000000000000 ) ) ;
#15014=CARTESIAN_POINT ( 'NONE',  ( 0.000000000000000000, 4.580371886574746102E-17, 0.3740157480314960647 ) ) ;
#15042=EDGE_CURVE ( 'NONE', #16233, #6811, #26987, .T. ) ;
#15045=ORIENTED_EDGE ( 'NONE', *, *, #3875, .T. ) ;
#15047=LINE ( 'NONE', #6153, #21589 ) ;
#15061=AXIS2_PLACEMENT_3D ( 'NONE', #21932, #19802, #17671 ) ;
#15064=DIRECTION ( 'NONE',  ( 1.000000000000000000, 0.000000000000000000, 0.000000000000000000 ) ) ;
#15104=CIRCLE ( 'NONE', #14645, 0.4941010236220472751 ) ;
#15116=CIRCLE ( 'NONE', #12833, 0.3740157480314960647 ) ;
#15130=CARTESIAN_POINT ( 'NONE',  ( 0.1516263115863346334, 0.1971492568089275588, 0.4530651079966787620 ) ) ;
#15144=DIRECTION ( 'NONE',  ( 1.000000000000000000, 0.000000000000000000, 0.000000000000000000 ) ) ;
#15145=CARTESIAN_POINT ( 'NONE',  ( 0.07614184848677874040, 0.4941010236220472751, 0.000000000000000000 ) ) ;
#15159=FACE_OUTER_BOUND ( 'NONE', #10192, .T. ) ;
#15174=AXIS2_PLACEMENT_3D ( 'NONE', #4576, #11210, #2455 ) ;
#15176=CARTESIAN_POINT ( 'NONE',  ( 0.1516263115863346334, 0.1971492568089271424, -0.4530651079966795947 ) ) ;
#15185=CONICAL_SURFACE ( 'NONE', #6180, 0.1106489370078740098, 0.08726646250000029414 ) ;
#15188=CARTESIAN_POINT ( 'NONE',  ( 0.5905511811023621549, 0.000000000000000000, -0.3346456692913385988 ) ) ;
#15209=CIRCLE ( 'NONE', #2982, 0.4941010236220472751 ) ;
#15219=CARTESIAN_POINT ( 'NONE',  ( 0.1518453843511950729, -0.2938239883646063255, 0.3972446186700991921 ) ) ;
#15228=B_SPLINE_CURVE_WITH_KNOTS ( 'NONE', 3,
 ( #20114, #11499, #773, #5131, #14481, #22946 ),
 .UNSPECIFIED., .F., .F.,
 ( 4, 2, 4 ),
 ( 4.334600841719497663E-14, 0.0007294371397779656667, 0.001458874279512585364 ),
 .UNSPECIFIED. ) ;
#15273=STYLED_ITEM ( 'NONE', ( #23350 ), #21416 ) ;
#15287=AXIS2_PLACEMENT_3D ( 'NONE', #20151, #26938, #20433 ) ;
#15296=VECTOR ( 'NONE', #17563, 39.37007874015748854 ) ;
#15303=DIRECTION ( 'NONE',  ( 1.000000000000000000, 0.000000000000000000, 0.000000000000000000 ) ) ;
#15314=CIRCLE ( 'NONE', #25656, 0.1298643763538141760 ) ;
#15323=AXIS2_PLACEMENT_3D ( 'NONE', #26196, #19841, #498 ) ;
#15324=FACE_OUTER_BOUND ( 'NONE', #18528, .T. ) ;
#15348=ORIENTED_EDGE ( 'NONE', *, *, #20542, .T. ) ;
#15350=EDGE_LOOP ( 'NONE', ( #16627, #20410, #18524, #19611, #7709, #4731, #4594, #26210, #14434, #22168, #18740, #18136, #23909, #14188, #25969, #22649 ) ) ;
#15369=VECTOR ( 'NONE', #24153, 39.37007874015748854 ) ;
#15371=ORIENTED_EDGE ( 'NONE', *, *, #4375, .F. ) ;
#15377=PLANE ( 'NONE',  #10425 ) ;
#15433=EDGE_CURVE ( 'NONE', #12691, #7184, #22782, .T. ) ;
#15443=VERTEX_POINT ( 'NONE', #8203 ) ;
#15469=DIRECTION ( 'NONE',  ( 0.000000000000000000, 1.000000000000000000, 0.000000000000000000 ) ) ;
#15470=VERTEX_POINT ( 'NONE', #27412 ) ;
#15488=CARTESIAN_POINT ( 'NONE',  ( 0.1522836969735573143, 0.000000000000000000, 0.000000000000000000 ) ) ;
#15498=EDGE_CURVE ( 'NONE', #18835, #4773, #5169, .T. ) ;
#15580=CARTESIAN_POINT ( 'NONE',  ( 0.1490609433576163545, -0.2393035190829114200, 0.4144858534816307505 ) ) ;
#15587=ADVANCED_FACE ( 'NONE', ( #18452 ), #9693, .F. ) ;
#15592=PLANE ( 'NONE',  #15751 ) ;
#15615=VERTEX_POINT ( 'NONE', #20737 ) ;
#15651=VERTEX_POINT ( 'NONE', #7638 ) ;
#15653=DIRECTION ( 'NONE',  ( 0.000000000000000000, 1.000000000000000000, -1.224646799147353207E-16 ) ) ;
#15656=EDGE_LOOP ( 'NONE', ( #14462, #5814, #27842, #5155 ) ) ;
#15672=CARTESIAN_POINT ( 'NONE',  ( 0.1522836969735573143, -0.4909267390297480382, 0.05591742528025181458 ) ) ;
#15678=ORIENTED_EDGE ( 'NONE', *, *, #6471, .F. ) ;
#15681=CARTESIAN_POINT ( 'NONE',  ( 0.1493295869868994930, 0.4796200322303180164, -0.01881014177756113945 ) ) ;
#15682=DIRECTION ( 'NONE',  ( 1.000000000000000000, 0.000000000000000000, 0.000000000000000000 ) ) ;
#15696=AXIS2_PLACEMENT_3D ( 'NONE', #5133, #1060, #2863 ) ;
#15697=DIRECTION ( 'NONE',  ( 1.000000000000000000, 0.000000000000000000, 0.000000000000000000 ) ) ;
#15701=ORIENTED_EDGE ( 'NONE', *, *, #3170, .T. ) ;
#15721=CARTESIAN_POINT ( 'NONE',  ( 0.3149606299212598381, -0.3346456692913385988, 4.098227477461615257E-17 ) ) ;
#15738=CIRCLE ( 'NONE', #15323, 0.4786070381542913421 ) ;
#15751=AXIS2_PLACEMENT_3D ( 'NONE', #22068, #11064, #19689 ) ;
#15759=EDGE_CURVE ( 'NONE', #13737, #11023, #21572, .T. ) ;
#15766=DIRECTION ( 'NONE',  ( -0.9790454724845842893, 0.2036417511401760472, 0.000000000000000000 ) ) ;
#15776=ORIENTED_EDGE ( 'NONE', *, *, #8388, .F. ) ;
#15778=ORIENTED_EDGE ( 'NONE', *, *, #665, .F. ) ;
#15812=CIRCLE ( 'NONE', #19427, 0.3346456692913385988 ) ;
#15832=DIRECTION ( 'NONE',  ( 1.000000000000000000, 0.000000000000000000, 0.000000000000000000 ) ) ;
#15864=CARTESIAN_POINT ( 'NONE',  ( 0.1755067523729419432, 0.3028750839302637998, 0.5245950337139047015 ) ) ;
#15876=DIRECTION ( 'NONE',  ( -0.2036417511401759084, 0.4895227362422917006, -0.8478782506317888989 ) ) ;
#15879=CARTESIAN_POINT ( 'NONE',  ( 0.5905511811023621549, 0.000000000000000000, 0.000000000000000000 ) ) ;
#15882=CARTESIAN_POINT ( 'NONE',  ( 0.3905379133858267737, 0.2805118110236220486, 0.4858607088160724063 ) ) ;
#15910=ORIENTED_EDGE ( 'NONE', *, *, #12178, .F. ) ;
#15921=VERTEX_POINT ( 'NONE', #20239 ) ;
#15928=CARTESIAN_POINT ( 'NONE',  ( 0.1522836969735573143, 0.1970374587079574968, -0.4531137400369417145 ) ) ;
#15937=ORIENTED_EDGE ( 'NONE', *, *, #8802, .F. ) ;
#15955=DIRECTION ( 'NONE',  ( 0.000000000000000000, 1.000000000000000000, 0.000000000000000000 ) ) ;
#15964=EDGE_CURVE ( 'NONE', #20796, #24033, #1158, .T. ) ;
#15995=FACE_OUTER_BOUND ( 'NONE', #5842, .T. ) ;
#16000=CARTESIAN_POINT ( 'NONE',  ( 0.1490609433615242285, 0.000000000000000000, 0.000000000000000000 ) ) ;
#16011=VECTOR ( 'NONE', #22821, 39.37007874015748854 ) ;
#16012=CIRCLE ( 'NONE', #26838, 0.09143349766193348271 ) ;
#16052=ORIENTED_EDGE ( 'NONE', *, *, #12492, .T. ) ;
#16080=EDGE_CURVE ( 'NONE', #5524, #4811, #24587, .T. ) ;
#16115=CARTESIAN_POINT ( 'NONE',  ( 0.1490609433615240342, -0.2393035190771456711, 0.4144858534716441278 ) ) ;
#16136=FACE_OUTER_BOUND ( 'NONE', #7059, .T. ) ;
#16156=AXIS2_PLACEMENT_3D ( 'NONE', #10696, #17197, #25816 ) ;
#16159=AXIS2_PLACEMENT_3D ( 'NONE', #15879, #3286, #24484 ) ;
#16161=FACE_OUTER_BOUND ( 'NONE', #26776, .T. ) ;
#16167=CARTESIAN_POINT ( 'NONE',  ( 0.1522836969735573143, -0.2938892803217901806, -0.3971963147566889840 ) ) ;
#16174=DIRECTION ( 'NONE',  ( 0.000000000000000000, -1.000000000000000000, 0.000000000000000000 ) ) ;
#16180=CIRCLE ( 'NONE', #19321, 0.4786070381542913421 ) ;
#16230=DIRECTION ( 'NONE',  ( 1.000000000000000000, 0.000000000000000000, 0.000000000000000000 ) ) ;
#16233=VERTEX_POINT ( 'NONE', #15580 ) ;
#16251=ORIENTED_EDGE ( 'NONE', *, *, #6742, .F. ) ;
#16273=FACE_OUTER_BOUND ( 'NONE', #24510, .T. ) ;
#16275=ORIENTED_EDGE ( 'NONE', *, *, #21382, .T. ) ;
#16288=CARTESIAN_POINT ( 'NONE',  ( 0.1516263115863346334, -0.4909405214979283838, 0.05579628926458630317 ) ) ;
#16305=CARTESIAN_POINT ( 'NONE',  ( 0.5925575908939920700, -0.2268709785195988371, 0.3929520615588126264 ) ) ;
#16322=VERTEX_POINT ( 'NONE', #593 ) ;
#16343=ADVANCED_FACE ( 'NONE', ( #2821 ), #13859, .T. ) ;
#16382=CARTESIAN_POINT ( 'NONE',  ( 0.1490609433615242285, 0.000000000000000000, 0.000000000000000000 ) ) ;
#16403=SURFACE_SIDE_STYLE ('',( #1851 ) ) ;
#16454=ADVANCED_FACE ( 'NONE', ( #12025 ), #4530, .T. ) ;
#16484=ORIENTED_EDGE ( 'NONE', *, *, #13842, .T. ) ;
#16488=DIRECTION ( 'NONE',  ( -0.9790454724845842893, 0.1018208755700880375, -0.1763589297585410332 ) ) ;
#16497=CARTESIAN_POINT ( 'NONE',  ( 0.1517511419331917244, -0.4888569460008191370, 0.05146517564439353348 ) ) ;
#16509=CARTESIAN_POINT ( 'NONE',  ( 0.1516263115863346334, 0.1971492568089271424, -0.4530651079966795947 ) ) ;
#16527=DIRECTION ( 'NONE',  ( 0.000000000000000000, 1.000000000000000000, 0.000000000000000000 ) ) ;
#16551=DIRECTION ( 'NONE',  ( 1.000000000000000000, 0.000000000000000000, 0.000000000000000000 ) ) ;
#16555=EDGE_LOOP ( 'NONE', ( #26358, #2697, #14315, #1650 ) ) ;
#16599=ORIENTED_EDGE ( 'NONE', *, *, #21466, .T. ) ;
#16610=VERTEX_POINT ( 'NONE', #2256 ) ;
#16612=CARTESIAN_POINT ( 'NONE',  ( 0.1490609433576163545, -0.2393035190829114200, 0.4144858534816307505 ) ) ;
#16617=CARTESIAN_POINT ( 'NONE',  ( 0.1490609433615240342, 0.2393035190771456711, 0.4144858534716441278 ) ) ;
#16627=ORIENTED_EDGE ( 'NONE', *, *, #8131, .T. ) ;
#16641=ORIENTED_EDGE ( 'NONE', *, *, #2816, .T. ) ;
#16668=CIRCLE ( 'NONE', #16156, 0.09143349766193348271 ) ;
#16673=DIRECTION ( 'NONE',  ( -0.9790454724845842893, 0.1018208755700880375, -0.1763589297585410332 ) ) ;
#16674=CIRCLE ( 'NONE', #9884, 0.4807043897637795493 ) ;
#16689=CARTESIAN_POINT ( 'NONE',  ( 0.3680051700917441604, 0.000000000000000000, 0.000000000000000000 ) ) ;
#16719=EDGE_CURVE ( 'NONE', #13737, #11023, #2664, .T. ) ;
#16742=CARTESIAN_POINT ( 'NONE',  ( 0.1522836969815822838, -0.2938892803218252081, 0.3971963147669425598 ) ) ;
#16759=CIRCLE ( 'NONE', #20823, 0.4941010236220472751 ) ;
#16762=DIRECTION ( 'NONE',  ( -0.2036417511401761582, -0.4895227362422917006, -0.8478782506317886769 ) ) ;
#16766=VECTOR ( 'NONE', #3015, 39.37007874015748854 ) ;
#16783=VERTEX_POINT ( 'NONE', #984 ) ;
#16790=ORIENTED_EDGE ( 'NONE', *, *, #25771, .T. ) ;
#16808=CARTESIAN_POINT ( 'NONE',  ( 0.1516263115863346334, -0.4909405214979283838, -0.05579628926458622684 ) ) ;
#16826=VECTOR ( 'NONE', #20964, 39.37007874015748143 ) ;
#16877=AXIS2_PLACEMENT_3D ( 'NONE', #20445, #3331, #7444 ) ;
#16924=ADVANCED_FACE ( 'NONE', ( #11498 ), #9360, .T. ) ;
#16926=DIRECTION ( 'NONE',  ( 0.2036417511401770464, 0.4895227362422922002, 0.8478782506317882328 ) ) ;
#16965=FACE_OUTER_BOUND ( 'NONE', #20141, .T. ) ;
#16972=CIRCLE ( 'NONE', #17403, 0.09143349766193348271 ) ;
#16984=EDGE_CURVE ( 'NONE', #16322, #13098, #4518, .T. ) ;
#16987=DIRECTION ( 'NONE',  ( 0.000000000000000000, 1.000000000000000000, 0.000000000000000000 ) ) ;
#16991=VECTOR ( 'NONE', #22028, 39.37007874015748143 ) ;
#17003=CARTESIAN_POINT ( 'NONE',  ( 0.6241887519799541595, -0.3029073140874564696, 0.5246508579836981490 ) ) ;
#17031=DIRECTION ( 'NONE',  ( 0.000000000000000000, 1.000000000000000000, 0.000000000000000000 ) ) ;
#17073=CARTESIAN_POINT ( 'NONE',  ( 0.5925575908939920700, 0.000000000000000000, 0.000000000000000000 ) ) ;
#17074=ORIENTED_EDGE ( 'NONE', *, *, #20391, .F. ) ;
#17110=EDGE_CURVE ( 'NONE', #16783, #6811, #27086, .T. ) ;
#17124=ORIENTED_EDGE ( 'NONE', *, *, #22693, .F. ) ;
#17185=AXIS2_PLACEMENT_3D ( 'NONE', #17873, #26366, #13506 ) ;
#17197=DIRECTION ( 'NONE',  ( -0.9790454724845842893, -0.1018208755700880375, -0.1763589297585410332 ) ) ;
#17206=VERTEX_POINT ( 'NONE', #14775 ) ;
#17211=ORIENTED_EDGE ( 'NONE', *, *, #27831, .F. ) ;
#17226=CARTESIAN_POINT ( 'NONE',  ( 0.1522836969735573143, 0.2938892803217905692, 0.3971963147566898167 ) ) ;
#17231=CARTESIAN_POINT ( 'NONE',  ( 0.1525037638700916243, 0.2637554987713724985, 0.4194810972668291393 ) ) ;
#17235=LINE ( 'NONE', #25432, #27439 ) ;
#17247=CARTESIAN_POINT ( 'NONE',  ( 0.1506723201675407575, 0.000000000000000000, 0.000000000000000000 ) ) ;
#17252=( BOUNDED_CURVE ( )  B_SPLINE_CURVE ( 3, ( #11614, #3263, #7671, #16288 ),
 .UNSPECIFIED., .F., .T. ) 
 B_SPLINE_CURVE_WITH_KNOTS ( ( 4, 4 ),
 ( 3.141592653589793116, 3.254758905499643973 ),
 .UNSPECIFIED. ) 
 CURVE ( )  GEOMETRIC_REPRESENTATION_ITEM ( )  RATIONAL_B_SPLINE_CURVE ( ( 1.000000000000000000, 0.9989330679932157953, 0.9989330679932157953, 1.000000000000000000 ) ) 
 REPRESENTATION_ITEM ( '' )  ) ;
#17262=CARTESIAN_POINT ( 'NONE',  ( 0.1522836969735573143, 0.000000000000000000, 0.000000000000000000 ) ) ;
#17270=EDGE_LOOP ( 'NONE', ( #12133, #25352, #11525, #11668 ) ) ;
#17275=VERTEX_POINT ( 'NONE', #23653 ) ;
#17279=DIRECTION ( 'NONE',  ( 0.000000000000000000, 1.000000000000000000, 0.000000000000000000 ) ) ;
#17280=DIRECTION ( 'NONE',  ( -0.2036417511401759362, -0.4895227362422912565, 0.8478782506317890100 ) ) ;
#17282=EDGE_CURVE ( 'NONE', #22329, #17815, #24146, .T. ) ;
#17283=CONICAL_SURFACE ( 'NONE', #17706, 0.1106489370078740930, 0.08726646250000029414 ) ;
#17306=CARTESIAN_POINT ( 'NONE',  ( 0.1518453844022533417, 0.1971119370939669324, -0.4530813475038473204 ) ) ;
#17323=ADVANCED_FACE ( 'NONE', ( #15324 ), #91, .T. ) ;
#17333=ADVANCED_FACE ( 'NONE', ( #13035 ), #25614, .T. ) ;
#17341=DIRECTION ( 'NONE',  ( -0.2036417511401759084, 0.4895227362422917006, -0.8478782506317888989 ) ) ;
#17346=ORIENTED_EDGE ( 'NONE', *, *, #27426, .F. ) ;
#17347=CARTESIAN_POINT ( 'NONE',  ( 0.1522836969735571200, -0.4941010236220468865, -0.01864847287710779539 ) ) ;
#17362=CARTESIAN_POINT ( 'NONE',  ( 0.1493402947442836470, -0.2564861316490620879, 0.4057730592017521065 ) ) ;
#17371=CIRCLE ( 'NONE', #6115, 0.3740157480314960647 ) ;
#17403=AXIS2_PLACEMENT_3D ( 'NONE', #18038, #3218, #26827 ) ;
#17408=ORIENTED_EDGE ( 'NONE', *, *, #9644, .T. ) ;
#17409=AXIS2_PLACEMENT_3D ( 'NONE', #25643, #10516, #17031 ) ;
#17411=CARTESIAN_POINT ( 'NONE',  ( 0.07614184848677874040, 0.000000000000000000, 0.000000000000000000 ) ) ;
#17433=DIRECTION ( 'NONE',  ( 1.000000000000000000, 0.000000000000000000, 0.000000000000000000 ) ) ;
#17448=CARTESIAN_POINT ( 'NONE',  ( 0.1522836969735573143, -0.2938892803217901806, -0.3971963147566889840 ) ) ;
#17450=ADVANCED_FACE ( 'NONE', ( #1706 ), #20782, .T. ) ;
#17471=CARTESIAN_POINT ( 'NONE',  ( 0.5981657849660177995, 0.4807043897637795493, 0.000000000000000000 ) ) ;
#17475=CARTESIAN_POINT ( 'NONE',  ( 0.1512183756282267089, 0.2841060247040496090, -0.3980637497190844809 ) ) ;
#17479=EDGE_LOOP ( 'NONE', ( #13534, #5894, #6147, #4782 ) ) ;
#17491=DIRECTION ( 'NONE',  ( -0.9790454724845842893, 0.2036417511401760472, 0.000000000000000000 ) ) ;
#17496=DIRECTION ( 'NONE',  ( -1.000000000000000000, 0.000000000000000000, 0.000000000000000000 ) ) ;
#17503=DIRECTION ( 'NONE',  ( 0.9790454724845839563, 0.1018208755700887314, 0.1763589297585421989 ) ) ;
#17544=DIRECTION ( 'NONE',  ( -0.9790454724845842893, -0.2036417511401760472, 2.493892000000000781E-17 ) ) ;
#17563=DIRECTION ( 'NONE',  ( -0.9575713608335526539, -0.1440981340193016325, -0.2495852893972989595 ) ) ;
#17581=ORIENTED_EDGE ( 'NONE', *, *, #25869, .F. ) ;
#17617=EDGE_LOOP ( 'NONE', ( #25888, #9529, #6974, #24977 ) ) ;
#17632=ADVANCED_FACE ( 'NONE', ( #11025 ), #8492, .F. ) ;
#17635=VERTEX_POINT ( 'NONE', #21630 ) ;
#17646=ORIENTED_EDGE ( 'NONE', *, *, #17751, .F. ) ;
#17652=FACE_OUTER_BOUND ( 'NONE', #3148, .T. ) ;
#17656=ADVANCED_FACE ( 'NONE', ( #26002 ), #11642, .T. ) ;
#17671=DIRECTION ( 'NONE',  ( 0.000000000000000000, 1.000000000000000000, 0.000000000000000000 ) ) ;
#17681=CARTESIAN_POINT ( 'NONE',  ( 0.4130706566799093316, -0.3346769814300175616, -0.5796775359605755851 ) ) ;
#17695=FACE_OUTER_BOUND ( 'NONE', #15350, .T. ) ;
#17706=AXIS2_PLACEMENT_3D ( 'NONE', #15882, #3427, #7260 ) ;
#17743=ORIENTED_EDGE ( 'NONE', *, *, #17751, .T. ) ;
#17751=EDGE_CURVE ( 'NONE', #22705, #4526, #14374, .T. ) ;
#17767=DIRECTION ( 'NONE',  ( -0.9790454724845842893, 0.1018208755700880375, 0.1763589297585410332 ) ) ;
#17778=CARTESIAN_POINT ( 'NONE',  ( 0.5869493968219645641, -0.2133897621573078718, -0.3696019098714952711 ) ) ;
#17795=CARTESIAN_POINT ( 'NONE',  ( 0.1520645003235147619, 0.2938566582844236441, 0.3972204521082409734 ) ) ;
#17815=VERTEX_POINT ( 'NONE', #16509 ) ;
#17854=EDGE_LOOP ( 'NONE', ( #18498, #10342, #1670 ) ) ;
#17873=CARTESIAN_POINT ( 'NONE',  ( 0.03937007874015747977, 0.000000000000000000, 0.000000000000000000 ) ) ;
#17895=CARTESIAN_POINT ( 'NONE',  ( 0.1522836969735573143, -0.4909267390297480382, -0.05591742528025173131 ) ) ;
#17901=CARTESIAN_POINT ( 'NONE',  ( 0.3905379133858267737, 0.2805118110236220486, -0.4858607088160732390 ) ) ;
#17902=CARTESIAN_POINT ( 'NONE',  ( 0.1490609433615242285, 0.4786070381542913421, 0.000000000000000000 ) ) ;
#17906=APPLICATION_CONTEXT ( 'automotive_design' ) ;
#17937=ORIENTED_EDGE ( 'NONE', *, *, #8260, .T. ) ;
#17959=CARTESIAN_POINT ( 'NONE',  ( 0.5905511811023621549, 4.339299682018180063E-17, 0.3346456692913385988 ) ) ;
#17994=ORIENTED_EDGE ( 'NONE', *, *, #21668, .F. ) ;
#18031=ORIENTED_EDGE ( 'NONE', *, *, #26551, .T. ) ;
#18038=CARTESIAN_POINT ( 'NONE',  ( 0.6055690743987126590, -0.2581485381169802973, 0.4471263839182408883 ) ) ;
#18055=CARTESIAN_POINT ( 'NONE',  ( 0.1525037638700916243, -0.2637554987713726651, -0.4194810972668291393 ) ) ;
#18060=DIRECTION ( 'NONE',  ( 1.000000000000000000, 0.000000000000000000, 0.000000000000000000 ) ) ;
#18062=CIRCLE ( 'NONE', #21725, 0.3346456692913385988 ) ;
#18112=( BOUNDED_CURVE ( )  B_SPLINE_CURVE ( 3, ( #2893, #20144, #17347, #8992 ),
 .UNSPECIFIED., .F., .F. ) 
 B_SPLINE_CURVE_WITH_KNOTS ( ( 4, 4 ),
 ( 3.028426401679942259, 3.141592653589793116 ),
 .UNSPECIFIED. ) 
 CURVE ( )  GEOMETRIC_REPRESENTATION_ITEM ( )  RATIONAL_B_SPLINE_CURVE ( ( 1.000000000000000000, 0.9989330679932157953, 0.9989330679932157953, 1.000000000000000000 ) ) 
 REPRESENTATION_ITEM ( '' )  ) ;
#18122=EDGE_CURVE ( 'NONE', #1802, #11062, #27445, .T. ) ;
#18136=ORIENTED_EDGE ( 'NONE', *, *, #615, .T. ) ;
#18163=AXIS2_PLACEMENT_3D ( 'NONE', #18570, #9537, #11812 ) ;
#18166=ORIENTED_EDGE ( 'NONE', *, *, #7420, .F. ) ;
#18173=AXIS2_PLACEMENT_3D ( 'NONE', #13497, #2625, #11250 ) ;
#18183=CARTESIAN_POINT ( 'NONE',  ( 0.1501355178992943018, 0.4826710871606305076, -0.03296692058268119868 ) ) ;
#18196=CARTESIAN_POINT ( 'NONE',  ( 0.1516263115863346334, 0.4909405214979283838, -0.05579628926458630317 ) ) ;
#18206=ORIENTED_EDGE ( 'NONE', *, *, #12492, .F. ) ;
#18210=VERTEX_POINT ( 'NONE', #27362 ) ;
#18212=CIRCLE ( 'NONE', #1114, 0.4267795243146149664 ) ;
#18232=CIRCLE ( 'NONE', #677, 0.1298643763538141760 ) ;
#18234=DIRECTION ( 'NONE',  ( 0.000000000000000000, -1.000000000000000000, 0.000000000000000000 ) ) ;
#18237=EDGE_CURVE ( 'NONE', #7963, #280, #10394, .T. ) ;
#18242=LENGTH_MEASURE_WITH_UNIT ( LENGTH_MEASURE( 0.02539999999999999897 ), #11764 ) ;
#18261=FACE_OUTER_BOUND ( 'NONE', #27492, .T. ) ;
#18265=AXIS2_PLACEMENT_3D ( 'NONE', #9168, #707, #26143 ) ;
#18302=FACE_OUTER_BOUND ( 'NONE', #7008, .T. ) ;
#18316=CARTESIAN_POINT ( 'NONE',  ( 0.5981657849660177995, 0.2403521948818893861, -0.4163022132461299263 ) ) ;
#18329=CARTESIAN_POINT ( 'NONE',  ( 0.5981657849660177995, 0.000000000000000000, 0.000000000000000000 ) ) ;
#18349=ORIENTED_EDGE ( 'NONE', *, *, #21190, .T. ) ;
#18359=EDGE_LOOP ( 'NONE', ( #15348, #22961 ) ) ;
#18365=AXIS2_PLACEMENT_3D ( 'NONE', #19416, #25778, #15469 ) ;
#18380=AXIS2_PLACEMENT_3D ( 'NONE', #17247, #15144, #12999 ) ;
#18381=ORIENTED_EDGE ( 'NONE', *, *, #6742, .T. ) ;
#18415=CARTESIAN_POINT ( 'NONE',  ( 0.6055690743987126590, 0.5162970762339605946, 0.000000000000000000 ) ) ;
#18452=FACE_OUTER_BOUND ( 'NONE', #6398, .T. ) ;
#18471=DIRECTION ( 'NONE',  ( 1.000000000000000000, 0.000000000000000000, 0.000000000000000000 ) ) ;
#18476=EDGE_CURVE ( 'NONE', #23841, #14598, #21625, .T. ) ;
#18498=ORIENTED_EDGE ( 'NONE', *, *, #1889, .F. ) ;
#18499=LENGTH_MEASURE_WITH_UNIT ( LENGTH_MEASURE( 0.02539999999999999897 ), #23197 ) ;
#18518=CARTESIAN_POINT ( 'NONE',  ( 0.5981657849660177995, -0.2403521948818897747, -0.4163022132461299263 ) ) ;
#18524=ORIENTED_EDGE ( 'NONE', *, *, #12030, .T. ) ;
#18528=EDGE_LOOP ( 'NONE', ( #7512, #9526, #19170, #8597, #18755, #3389, #5571, #11108, #413, #10583, #15045, #4068, #17937, #15937, #12844, #5869 ) ) ;
#18530=CARTESIAN_POINT ( 'NONE',  ( 0.2019525613798653640, -0.7328932975451569742, 7.384975690285532084E-17 ) ) ;
#18531=ORIENTED_EDGE ( 'NONE', *, *, #15498, .T. ) ;
#18538=AXIS2_PLACEMENT_3D ( 'NONE', #16689, #27711, #12298 ) ;
#18543=DIRECTION ( 'NONE',  ( -0.2036417511401760472, -0.4895227362422912565, 0.8478782506317888989 ) ) ;
#18545=EDGE_CURVE ( 'NONE', #24440, #3752, #9810, .T. ) ;
#18570=CARTESIAN_POINT ( 'NONE',  ( 0.5925575908939920700, -0.4537419570391968415, 5.556736220472441090E-17 ) ) ;
#18604=CARTESIAN_POINT ( 'NONE',  ( 0.1504778549387067454, -0.4839706879307174581, 0.03773480285810273255 ) ) ;
#18650=ORIENTED_EDGE ( 'NONE', *, *, #22693, .T. ) ;
#18684=CARTESIAN_POINT ( 'NONE',  ( 0.1493967478962657525, 0.4798749592428784849, 0.01883130896441918486 ) ) ;
#18703=ORIENTED_EDGE ( 'NONE', *, *, #21085, .T. ) ;
#18707=ADVANCED_FACE ( 'NONE', ( #10003 ), #4502, .F. ) ;
#18710=CARTESIAN_POINT ( 'NONE',  ( 0.5925575908939920700, 0.000000000000000000, 0.000000000000000000 ) ) ;
#18740=ORIENTED_EDGE ( 'NONE', *, *, #1889, .T. ) ;
#18743=DIRECTION ( 'NONE',  ( 1.000000000000000000, 0.000000000000000000, 0.000000000000000000 ) ) ;
#18755=ORIENTED_EDGE ( 'NONE', *, *, #24031, .T. ) ;
#18758=VERTEX_POINT ( 'NONE', #7321 ) ;
#18788=( NAMED_UNIT ( * ) SI_UNIT ( $, .STERADIAN. ) SOLID_ANGLE_UNIT ( ) ) ;
#18803=CARTESIAN_POINT ( 'NONE',  ( 0.5869493968219645641, 0.000000000000000000, 0.000000000000000000 ) ) ;
#18814=LINE ( 'NONE', #5846, #12009 ) ;
#18830=ORIENTED_EDGE ( 'NONE', *, *, #8358, .T. ) ;
#18835=VERTEX_POINT ( 'NONE', #17959 ) ;
#18878=CARTESIAN_POINT ( 'NONE',  ( 0.000000000000000000, 0.4143733464566928815, 0.000000000000000000 ) ) ;
#18883=CIRCLE ( 'NONE', #27026, 0.4941010236220472751 ) ;
#18949=DIRECTION ( 'NONE',  ( -0.2036417511401760472, 0.4895227362422920336, 0.8478782506317883438 ) ) ;
#18987=EDGE_LOOP ( 'NONE', ( #23334, #20984, #3795, #16599 ) ) ;
#19007=DIRECTION ( 'NONE',  ( 0.2036417511401769909, 0.4895227362422910344, -0.8478782506317890100 ) ) ;
#19026=PLANE ( 'NONE',  #8890 ) ;
#19063=DIRECTION ( 'NONE',  ( 0.2036417511401769909, -0.4895227362422910344, 0.8478782506317890100 ) ) ;
#19076=ORIENTED_EDGE ( 'NONE', *, *, #25037, .F. ) ;
#19090=DIRECTION ( 'NONE',  ( 0.000000000000000000, 1.000000000000000000, 0.000000000000000000 ) ) ;
#19113=DIRECTION ( 'NONE',  ( 0.000000000000000000, 1.000000000000000000, 0.000000000000000000 ) ) ;
#19114=CARTESIAN_POINT ( 'NONE',  ( 0.03937007874015747977, 0.000000000000000000, 0.000000000000000000 ) ) ;
#19115=AXIS2_PLACEMENT_3D ( 'NONE', #25701, #21187, #14849 ) ;
#19131=ORIENTED_EDGE ( 'NONE', *, *, #15433, .F. ) ;
#19133=FACE_OUTER_BOUND ( 'NONE', #22066, .T. ) ;
#19139=ORIENTED_EDGE ( 'NONE', *, *, #20896, .T. ) ;
#19150=DIRECTION ( 'NONE',  ( 1.000000000000000000, 0.000000000000000000, 0.000000000000000000 ) ) ;
#19170=ORIENTED_EDGE ( 'NONE', *, *, #8862, .T. ) ;
#19173=EDGE_CURVE ( 'NONE', #12205, #15615, #15209, .T. ) ;
#19194=CARTESIAN_POINT ( 'NONE',  ( 0.1493967478962657525, -0.2236290876712151154, -0.4249995598268396790 ) ) ;
#19217=ORIENTED_EDGE ( 'NONE', *, *, #23660, .F. ) ;
#19299=TOROIDAL_SURFACE ( 'NONE', #16159, 0.3740157480314960647, 0.03937007874015747977 ) ;
#19321=AXIS2_PLACEMENT_3D ( 'NONE', #16000, #7518, #7105 ) ;
#19415=CARTESIAN_POINT ( 'NONE',  ( 0.1638952246732497953, 0.2749627978706437048, 0.4762495361032464958 ) ) ;
#19416=CARTESIAN_POINT ( 'NONE',  ( 0.1506723201675407575, 0.000000000000000000, 0.000000000000000000 ) ) ;
#19422=ORIENTED_EDGE ( 'NONE', *, *, #5522, .F. ) ;
#19427=AXIS2_PLACEMENT_3D ( 'NONE', #10055, #25035, #18234 ) ;
#19438=ORIENTED_EDGE ( 'NONE', *, *, #25037, .T. ) ;
#19440=( BOUNDED_CURVE ( )  B_SPLINE_CURVE ( 3, ( #20636, #25150, #1288, #10309 ),
 .UNSPECIFIED., .F., .F. ) 
 B_SPLINE_CURVE_WITH_KNOTS ( ( 4, 4 ),
 ( 6.170019055269735375, 6.283185307179586232 ),
 .UNSPECIFIED. ) 
 CURVE ( )  GEOMETRIC_REPRESENTATION_ITEM ( )  RATIONAL_B_SPLINE_CURVE ( ( 1.000000000000000000, 0.9989330679932157953, 0.9989330679932157953, 1.000000000000000000 ) ) 
 REPRESENTATION_ITEM ( '' )  ) ;
#19441=VECTOR ( 'NONE', #16926, 39.37007874015748854 ) ;
#19499=AXIS2_PLACEMENT_3D ( 'NONE', #22037, #21906, #2798 ) ;
#19562=AXIS2_PLACEMENT_3D ( 'NONE', #13529, #17503, #24405 ) ;
#19566=DIRECTION ( 'NONE',  ( -0.2036417511401759084, -0.4895227362422917006, -0.8478782506317888989 ) ) ;
#19567=EDGE_CURVE ( 'NONE', #25542, #19740, #25985, .T. ) ;
#19586=CARTESIAN_POINT ( 'NONE',  ( 0.1516263115863346334, -0.1971492568089271424, 0.4530651079966787620 ) ) ;
#19593=CARTESIAN_POINT ( 'NONE',  ( 0.3680051700917442714, 0.4526932812344531265, 0.000000000000000000 ) ) ;
#19596=VERTEX_POINT ( 'NONE', #4037 ) ;
#19611=ORIENTED_EDGE ( 'NONE', *, *, #18545, .T. ) ;
#19631=CARTESIAN_POINT ( 'NONE',  ( 0.5905511811023621549, 0.000000000000000000, 0.000000000000000000 ) ) ;
#19634=CARTESIAN_POINT ( 'NONE',  ( 0.1525037638700916243, 0.2314035372547589564, 0.4381595109572584690 ) ) ;
#19643=ORIENTED_EDGE ( 'NONE', *, *, #15498, .F. ) ;
#19645=VERTEX_POINT ( 'NONE', #21271 ) ;
#19650=DIRECTION ( 'NONE',  ( -0.2036417511401762970, 0.9790454724845841783, -1.198984999999999849E-16 ) ) ;
#19655=AXIS2_PLACEMENT_3D ( 'NONE', #24336, #13596, #4980 ) ;
#19668=ORIENTED_EDGE ( 'NONE', *, *, #3641, .F. ) ;
#19677=ORIENTED_EDGE ( 'NONE', *, *, #22246, .F. ) ;
#19689=DIRECTION ( 'NONE',  ( -0.1772802999855984940, 0.000000000000000000, 0.9841604011730080703 ) ) ;
#19706=CARTESIAN_POINT ( 'NONE',  ( 0.1520645003235147619, 0.1970746732862649619, -0.4530975571996346818 ) ) ;
#19740=VERTEX_POINT ( 'NONE', #246 ) ;
#19745=EDGE_CURVE ( 'NONE', #15470, #3752, #25065, .T. ) ;
#19752=ADVANCED_FACE ( 'NONE', ( #23676 ), #11532, .T. ) ;
#19753=CARTESIAN_POINT ( 'NONE',  ( 0.1522836969735573143, -0.1970374587079582740, -0.4531137400369409374 ) ) ;
#19765=VERTEX_POINT ( 'NONE', #19832 ) ;
#19768=DIRECTION ( 'NONE',  ( 0.000000000000000000, 1.000000000000000000, 0.000000000000000000 ) ) ;
#19786=AXIS2_PLACEMENT_3D ( 'NONE', #19114, #1605, #10209 ) ;
#19802=DIRECTION ( 'NONE',  ( 1.000000000000000000, 0.000000000000000000, 0.000000000000000000 ) ) ;
#19832=CARTESIAN_POINT ( 'NONE',  ( 0.2019525613798653640, 0.3664466487725785426, 0.6347042139374529102 ) ) ;
#19841=DIRECTION ( 'NONE',  ( 1.000000000000000000, 0.000000000000000000, 0.000000000000000000 ) ) ;
#19849=PLANE ( 'NONE',  #10714 ) ;
#19879=ADVANCED_FACE ( 'NONE', ( #13743 ), #7532, .F. ) ;
#19882=DIRECTION ( 'NONE',  ( 0.000000000000000000, 1.224646799147353700E-16, 1.000000000000000000 ) ) ;
#19888=ORIENTED_EDGE ( 'NONE', *, *, #17110, .F. ) ;
#19889=ADVANCED_FACE ( 'NONE', ( #7387 ), #15185, .T. ) ;
#19905=ORIENTED_EDGE ( 'NONE', *, *, #8131, .F. ) ;
#19923=CARTESIAN_POINT ( 'NONE',  ( 0.4130706566799093316, 0.3346769814300175061, -0.5796775359605764733 ) ) ;
#19938=DIRECTION ( 'NONE',  ( 1.000000000000000000, 0.000000000000000000, 0.000000000000000000 ) ) ;
#19952=CIRCLE ( 'NONE', #18173, 0.1298643763538141760 ) ;
#19973=ORIENTED_EDGE ( 'NONE', *, *, #26244, .F. ) ;
#19977=ADVANCED_FACE ( 'NONE', ( #10482 ), #13369, .T. ) ;
#19999=TOROIDAL_SURFACE ( 'NONE', #16877, 0.3740157480314960647, 0.03937007874015747977 ) ;
#20004=CARTESIAN_POINT ( 'NONE',  ( 0.1490609433615242285, 0.2393035190771452825, -0.4144858534716441278 ) ) ;
#20018=EDGE_CURVE ( 'NONE', #16610, #11062, #18814, .T. ) ;
#20052=DIRECTION ( 'NONE',  ( -0.2036417511401762970, -0.9790454724845841783, 0.000000000000000000 ) ) ;
#20077=EDGE_LOOP ( 'NONE', ( #1725, #9676, #4747, #3926, #1372, #11602 ) ) ;
#20096=CIRCLE ( 'NONE', #7934, 0.09143349766193348271 ) ;
#20112=CARTESIAN_POINT ( 'NONE',  ( 0.03937007874015747977, 0.000000000000000000, -0.3346456692913385988 ) ) ;
#20114=CARTESIAN_POINT ( 'NONE',  ( 0.1490609433576163545, 0.2393035190829114200, 0.4144858534816307505 ) ) ;
#20117=FACE_OUTER_BOUND ( 'NONE', #18359, .T. ) ;
#20119=AXIS2_PLACEMENT_3D ( 'NONE', #11148, #24412, #19768 ) ;
#20125=( BOUNDED_CURVE ( )  B_SPLINE_CURVE ( 3, ( #25603, #21506, #1723, #8231 ),
 .UNSPECIFIED., .F., .F. ) 
 B_SPLINE_CURVE_WITH_KNOTS ( ( 4, 4 ),
 ( 3.028426401679941815, 3.254758905499644417 ),
 .UNSPECIFIED. ) 
 CURVE ( )  GEOMETRIC_REPRESENTATION_ITEM ( )  RATIONAL_B_SPLINE_CURVE ( ( 1.000000000000000000, 0.9957356870045845909, 0.9957356870045845909, 1.000000000000000000 ) ) 
 REPRESENTATION_ITEM ( '' )  ) ;
#20130=DIRECTION ( 'NONE',  ( -0.9930684569432060016, 0.1175373975568611284, 0.000000000000000000 ) ) ;
#20141=EDGE_LOOP ( 'NONE', ( #2417, #6885, #10431, #3171, #17581, #22096 ) ) ;
#20144=CARTESIAN_POINT ( 'NONE',  ( 0.1520643344662694629, -0.4930463976998556985, -0.03726710077533015864 ) ) ;
#20151=CARTESIAN_POINT ( 'NONE',  ( 0.1755067523729419432, -0.6057501678605275997, 7.418299212598425247E-17 ) ) ;
#20159=CIRCLE ( 'NONE', #6659, 0.09143349766193348271 ) ;
#20239=CARTESIAN_POINT ( 'NONE',  ( 0.1516263115863346334, -0.1971492568089275588, -0.4530651079966787620 ) ) ;
#20243=DIRECTION ( 'NONE',  ( 0.000000000000000000, 1.000000000000000000, 0.000000000000000000 ) ) ;
#20266=DIRECTION ( 'NONE',  ( 0.000000000000000000, 1.000000000000000000, 0.000000000000000000 ) ) ;
#20391=EDGE_CURVE ( 'NONE', #9781, #11452, #26990, .T. ) ;
#20395=DIRECTION ( 'NONE',  ( 0.000000000000000000, -0.8660254037844384856, -0.5000000000000003331 ) ) ;
#20402=CARTESIAN_POINT ( 'NONE',  ( 0.6140435224042697371, -0.4807043897637795493, 5.886930922602943265E-17 ) ) ;
#20403=PRODUCT_DEFINITION_CONTEXT ( 'detailed design', #17906, 'design' ) ;
#20406=EDGE_CURVE ( 'NONE', #15921, #17635, #14430, .T. ) ;
#20410=ORIENTED_EDGE ( 'NONE', *, *, #6931, .T. ) ;
#20422=FACE_OUTER_BOUND ( 'NONE', #17617, .T. ) ;
#20433=DIRECTION ( 'NONE',  ( -0.2036417511401760472, 0.9790454724845840673, -1.198985000000000095E-16 ) ) ;
#20440=DIRECTION ( 'NONE',  ( -0.9790454724845839563, 0.1018208755700880236, -0.1763589297585420324 ) ) ;
#20445=CARTESIAN_POINT ( 'NONE',  ( 0.5905511811023621549, 0.000000000000000000, 0.000000000000000000 ) ) ;
#20450=DIRECTION ( 'NONE',  ( -0.2036417511401760472, -0.9790454724845840673, 0.000000000000000000 ) ) ;
#20481=CARTESIAN_POINT ( 'NONE',  ( 0.5869493968219645641, 0.000000000000000000, 0.000000000000000000 ) ) ;
#20487=CARTESIAN_POINT ( 'NONE',  ( 0.1504127680534924905, -0.4837205684772389880, -0.03783905811610011050 ) ) ;
#20501=CARTESIAN_POINT ( 'NONE',  ( 0.6140435224042697371, 0.4807043897637795493, 0.000000000000000000 ) ) ;
#20523=CARTESIAN_POINT ( 'NONE',  ( 0.1516263115863346334, -0.4909405214979283838, -0.05579628926458622684 ) ) ;
#20538=DIRECTION ( 'NONE',  ( 1.000000000000000000, 0.000000000000000000, 0.000000000000000000 ) ) ;
#20540=CARTESIAN_POINT ( 'NONE',  ( 0.1512365935307563858, -0.2025838097703629714, 0.4452123804180691535 ) ) ;
#20542=EDGE_CURVE ( 'NONE', #21365, #11054, #2612, .T. ) ;
#20565=EDGE_CURVE ( 'NONE', #12967, #19645, #19440, .T. ) ;
#20585=CARTESIAN_POINT ( 'NONE',  ( 0.1522836969815822838, 0.1970374587168192970, 0.4531137400420984229 ) ) ;
#20586=CARTESIAN_POINT ( 'NONE',  ( 0.1518453843511950729, -0.1971119371026653633, -0.4530813475000614599 ) ) ;
#20605=EDGE_LOOP ( 'NONE', ( #12039, #25398, #9653, #18650, #19643, #6238 ) ) ;
#20616=DIRECTION ( 'NONE',  ( 1.000000000000000000, 0.000000000000000000, 0.000000000000000000 ) ) ;
#20636=CARTESIAN_POINT ( 'NONE',  ( 0.1516263115863346334, 0.4909405214979283838, 0.05579628926458630317 ) ) ;
#20641=EDGE_LOOP ( 'NONE', ( #25265, #5019 ) ) ;
#20678=CARTESIAN_POINT ( 'NONE',  ( 0.2019525613798654196, 0.3664466487725783206, -0.6347042139374537983 ) ) ;
#20684=VECTOR ( 'NONE', #24944, 39.37007874015748854 ) ;
#20737=CARTESIAN_POINT ( 'NONE',  ( 0.1522836969735573143, -0.1970374587079578854, 0.4531137400369409374 ) ) ;
#20743=ORIENTED_EDGE ( 'NONE', *, *, #23215, .F. ) ;
#20762=DIRECTION ( 'NONE',  ( 0.000000000000000000, 1.000000000000000000, 0.000000000000000000 ) ) ;
#20782=PLANE ( 'NONE',  #7553 ) ;
#20796=VERTEX_POINT ( 'NONE', #22548 ) ;
#20797=DIRECTION ( 'NONE',  ( 0.9930684569549264040, -0.05876869872891801738, -0.1017903720931950112 ) ) ;
#20804=CARTESIAN_POINT ( 'NONE',  ( 0.3680051700917441604, 0.000000000000000000, 0.000000000000000000 ) ) ;
#20818=CARTESIAN_POINT ( 'NONE',  ( 0.1522836969735572310, 0.4941010236220472751, 0.000000000000000000 ) ) ;
#20823=AXIS2_PLACEMENT_3D ( 'NONE', #23234, #4149, #25621 ) ;
#20834=ORIENTED_EDGE ( 'NONE', *, *, #20018, .F. ) ;
#20849=DIRECTION ( 'NONE',  ( -0.9930684569549264040, 0.05876869872891801738, -0.1017903720931950112 ) ) ;
#20880=FACE_OUTER_BOUND ( 'NONE', #2151, .T. ) ;
#20890=AXIS2_PLACEMENT_3D ( 'NONE', #22729, #20616, #23026 ) ;
#20896=EDGE_CURVE ( 'NONE', #17275, #16233, #15738, .T. ) ;
#20910=AXIS2_PLACEMENT_3D ( 'NONE', #5097, #7098, #13719 ) ;
#20937=AXIS2_PLACEMENT_3D ( 'NONE', #1828, #7775, #8337 ) ;
#20952=EDGE_CURVE ( 'NONE', #17815, #4811, #1606, .T. ) ;
#20964=DIRECTION ( 'NONE',  ( -0.9575713608335526539, -0.1440981340193014659, 0.2495852893972990150 ) ) ;
#20984=ORIENTED_EDGE ( 'NONE', *, *, #5093, .F. ) ;
#20999=DIRECTION ( 'NONE',  ( -0.9790454724845842893, 0.1018208755700882318, 0.1763589297585410332 ) ) ;
#21046=VERTEX_POINT ( 'NONE', #5565 ) ;
#21085=EDGE_CURVE ( 'NONE', #11452, #23841, #16674, .T. ) ;
#21099=CARTESIAN_POINT ( 'NONE',  ( 0.5869493968219645641, 0.000000000000000000, 0.000000000000000000 ) ) ;
#21106=VERTEX_POINT ( 'NONE', #17003 ) ;
#21113=ORIENTED_EDGE ( 'NONE', *, *, #27089, .F. ) ;
#21172=ORIENTED_EDGE ( 'NONE', *, *, #6354, .F. ) ;
#21180=ORIENTED_EDGE ( 'NONE', *, *, #11293, .F. ) ;
#21187=DIRECTION ( 'NONE',  ( 0.9790454724845839563, -0.1018208755700887314, -0.1763589297585421989 ) ) ;
#21190=EDGE_CURVE ( 'NONE', #22807, #11452, #3712, .T. ) ;
#21211=DIRECTION ( 'NONE',  ( 1.000000000000000000, 0.000000000000000000, 0.000000000000000000 ) ) ;
#21246=DIRECTION ( 'NONE',  ( 1.000000000000000000, 0.000000000000000000, 0.000000000000000000 ) ) ;
#21249=LINE ( 'NONE', #12344, #16826 ) ;
#21264=FACE_OUTER_BOUND ( 'NONE', #2205, .T. ) ;
#21267=AXIS2_PLACEMENT_3D ( 'NONE', #7332, #3072, #5354 ) ;
#21271=CARTESIAN_POINT ( 'NONE',  ( 0.1522836969735572310, 0.4941010236220472751, 0.000000000000000000 ) ) ;
#21277=DIRECTION ( 'NONE',  ( 0.9930684569549264040, 0.05876869872891801738, -0.1017903720931950112 ) ) ;
#21285=DIRECTION ( 'NONE',  ( 0.000000000000000000, 1.000000000000000000, 0.000000000000000000 ) ) ;
#21299=EDGE_CURVE ( 'NONE', #15651, #22705, #13432, .T. ) ;
#21330=PLANE ( 'NONE',  #19115 ) ;
#21349=CONICAL_SURFACE ( 'NONE', #12742, 0.4537419570391968415, 1.365720138124999927 ) ;
#21359=DIRECTION ( 'NONE',  ( 0.000000000000000000, 0.000000000000000000, -1.000000000000000000 ) ) ;
#21365=VERTEX_POINT ( 'NONE', #5533 ) ;
#21368=CIRCLE ( 'NONE', #11406, 0.4267795243146149664 ) ;
#21382=EDGE_CURVE ( 'NONE', #4526, #21365, #22480, .T. ) ;
#21416=MANIFOLD_SOLID_BREP ( 'Bearing Cone', #13694 ) ;
#21425=DIRECTION ( 'NONE',  ( -1.000000000000000000, 0.000000000000000000, 0.000000000000000000 ) ) ;
#21453=EDGE_LOOP ( 'NONE', ( #26779, #8727, #10603, #15678, #9187, #19677 ) ) ;
#21466=EDGE_CURVE ( 'NONE', #11023, #25542, #5497, .T. ) ;
#21472=CARTESIAN_POINT ( 'NONE',  ( 0.3680051700917442714, -0.4526932812344531265, 5.543894897734252589E-17 ) ) ;
#21476=CARTESIAN_POINT ( 'NONE',  ( 0.1516263115863346334, 0.2937912646890007973, 0.3972688187320929099 ) ) ;
#21506=CARTESIAN_POINT ( 'NONE',  ( 0.1525037638700916243, -0.2637554987713725541, 0.4194810972668290283 ) ) ;
#21520=ORIENTED_EDGE ( 'NONE', *, *, #24031, .F. ) ;
#21523=CARTESIAN_POINT ( 'NONE',  ( 0.6055690743987126590, 0.2581485381169799642, -0.4471263839182408883 ) ) ;
#21548=CARTESIAN_POINT ( 'NONE',  ( 0.1520645003235147619, -0.1970746732862649619, 0.4530975571996339046 ) ) ;
#21566=VERTEX_POINT ( 'NONE', #24014 ) ;
#21567=VECTOR ( 'NONE', #18060, 39.37007874015748143 ) ;
#21572=LINE ( 'NONE', #2208, #16011 ) ;
#21589=VECTOR ( 'NONE', #22879, 39.37007874015748854 ) ;
#21594=CARTESIAN_POINT ( 'NONE',  ( 0.5905511811023621549, -0.3346456692913385988, 4.098227477461615257E-17 ) ) ;
#21625=CIRCLE ( 'NONE', #26552, 0.4807043897637795493 ) ;
#21630=CARTESIAN_POINT ( 'NONE',  ( 0.1516263115863346334, -0.2937912646890007973, -0.3972688187320929099 ) ) ;
#21632=CARTESIAN_POINT ( 'NONE',  ( 0.1522836969735571200, 0.4941010236220468865, -0.01864847287710777804 ) ) ;
#21664=VECTOR ( 'NONE', #18471, 39.37007874015748143 ) ;
#21668=EDGE_CURVE ( 'NONE', #22807, #21106, #10897, .T. ) ;
#21676=ORIENTED_EDGE ( 'NONE', *, *, #13114, .F. ) ;
#21683=AXIS2_PLACEMENT_3D ( 'NONE', #22415, #15653, #19882 ) ;
#21709=ORIENTED_EDGE ( 'NONE', *, *, #2816, .F. ) ;
#21715=ORIENTED_EDGE ( 'NONE', *, *, #20565, .F. ) ;
#21725=AXIS2_PLACEMENT_3D ( 'NONE', #24350, #24483, #2861 ) ;
#21748=ADVANCED_FACE ( 'NONE', ( #7193 ), #26666, .T. ) ;
#21818=DIRECTION ( 'NONE',  ( 0.000000000000000000, 1.000000000000000000, 0.000000000000000000 ) ) ;
#21836=CARTESIAN_POINT ( 'NONE',  ( 0.1522836969735573143, 0.2938892803217905692, 0.3971963147566898167 ) ) ;
#21856=ADVANCED_FACE ( 'NONE', ( #519 ), #15377, .T. ) ;
#21863=CARTESIAN_POINT ( 'NONE',  ( 0.5869493968174713805, 0.4267795242930089161, 0.000000000000000000 ) ) ;
#21888=VERTEX_POINT ( 'NONE', #9818 ) ;
#21906=DIRECTION ( 'NONE',  ( -0.9790454724845842893, -0.1018208755700882318, 0.1763589297585410332 ) ) ;
#21922=EDGE_CURVE ( 'NONE', #16783, #23339, #20159, .T. ) ;
#21928=CARTESIAN_POINT ( 'NONE',  ( 0.6055690743987126590, -0.5162970762339605946, 6.322814960629921339E-17 ) ) ;
#21932=CARTESIAN_POINT ( 'NONE',  ( 0.5981657849660177995, 0.000000000000000000, 0.000000000000000000 ) ) ;
#22028=DIRECTION ( 'NONE',  ( 0.2036417511401760472, 0.9790454724845841783, 0.000000000000000000 ) ) ;
#22037=CARTESIAN_POINT ( 'NONE',  ( 0.3905379133858267737, -0.2805118110236220486, 0.4858607088160724063 ) ) ;
#22065=ADVANCED_FACE ( 'NONE', ( #21264 ), #2593, .F. ) ;
#22066=EDGE_LOOP ( 'NONE', ( #26125, #21113, #8140, #3647 ) ) ;
#22068=CARTESIAN_POINT ( 'NONE',  ( 0.1638952246732497953, -0.2749627978706437048, -0.4762495361032456631 ) ) ;
#22096=ORIENTED_EDGE ( 'NONE', *, *, #15759, .F. ) ;
#22106=DIRECTION ( 'NONE',  ( 1.000000000000000000, 0.000000000000000000, 0.000000000000000000 ) ) ;
#22109=ORIENTED_EDGE ( 'NONE', *, *, #4559, .T. ) ;
#22146=CARTESIAN_POINT ( 'NONE',  ( 0.1522836969735573143, -0.1970374587079582740, -0.4531137400369409374 ) ) ;
#22168=ORIENTED_EDGE ( 'NONE', *, *, #6354, .T. ) ;
#22221=( NAMED_UNIT ( * ) PLANE_ANGLE_UNIT ( ) SI_UNIT ( $, .RADIAN. ) ) ;
#22240=DIRECTION ( 'NONE',  ( 0.9790454724845840673, -0.1018208755700883150, 0.1763589297585418658 ) ) ;
#22246=EDGE_CURVE ( 'NONE', #19765, #12438, #6674, .T. ) ;
#22285=DIRECTION ( 'NONE',  ( -0.9930684569432060016, 0.05876869877843025891, -0.1017903721789531202 ) ) ;
#22298=LINE ( 'NONE', #11421, #16991 ) ;
#22320=EDGE_CURVE ( 'NONE', #6811, #11452, #17235, .T. ) ;
#22323=B_SPLINE_CURVE_WITH_KNOTS ( 'NONE', 3,
 ( #11567, #13687, #22448, #26676, #18183, #15681, #11997, #17902 ),
 .UNSPECIFIED., .F., .F.,
 ( 4, 2, 2, 4 ),
 ( 0.000000000000000000, 0.2499999999999998890, 0.4999999999999997780, 1.000000000000000000 ),
 .UNSPECIFIED. ) ;
#22329=VERTEX_POINT ( 'NONE', #22779 ) ;
#22334=B_SPLINE_CURVE_WITH_KNOTS ( 'NONE', 3,
 ( #24764, #20540, #3283, #7690, #7254, #11776 ),
 .UNSPECIFIED., .F., .F.,
 ( 4, 2, 4 ),
 ( 8.211396612100036608E-14, 0.0007294428068852505231, 0.001458885613688387043 ),
 .UNSPECIFIED. ) ;
#22366=CARTESIAN_POINT ( 'NONE',  ( 0.3149606299212598381, 0.000000000000000000, 0.000000000000000000 ) ) ;
#22368=DIRECTION ( 'NONE',  ( -0.9790454724845842893, -0.2036417511401760472, 2.493892000000000781E-17 ) ) ;
#22384=ORIENTED_EDGE ( 'NONE', *, *, #4559, .F. ) ;
#22385=FACE_OUTER_BOUND ( 'NONE', #5231, .T. ) ;
#22397=ORIENTED_EDGE ( 'NONE', *, *, #13838, .T. ) ;
#22400=AXIS2_PLACEMENT_3D ( 'NONE', #17073, #10559, #6210 ) ;
#22415=CARTESIAN_POINT ( 'NONE',  ( 0.03937007874015747977, 4.580371886574746102E-17, 0.3740157480314960647 ) ) ;
#22447=AXIS2_PLACEMENT_3D ( 'NONE', #22506, #11761, #13740 ) ;
#22448=CARTESIAN_POINT ( 'NONE',  ( 0.1512834625132478961, 0.4870552862735379462, -0.04694520391020851752 ) ) ;
#22480=LINE ( 'NONE', #20501, #21567 ) ;
#22496=DIRECTION ( 'NONE',  ( 0.000000000000000000, 0.000000000000000000, 1.000000000000000000 ) ) ;
#22501=CIRCLE ( 'NONE', #1294, 0.1298643763538141760 ) ;
#22506=CARTESIAN_POINT ( 'NONE',  ( 0.1755067523729419432, 0.3028750839302637998, 0.5245950337139047015 ) ) ;
#22521=EDGE_CURVE ( 'NONE', #23339, #280, #6002, .T. ) ;
#22546=EDGE_LOOP ( 'NONE', ( #3914, #6008, #6436, #23185, #12503, #563 ) ) ;
#22548=CARTESIAN_POINT ( 'NONE',  ( 0.6299212598425196763, 4.580371886574746102E-17, 0.3740157480314960647 ) ) ;
#22575=CARTESIAN_POINT ( 'NONE',  ( 0.1490609433615240342, 0.4786070381542913421, 0.000000000000000000 ) ) ;
#22586=ADVANCED_FACE ( 'NONE', ( #688 ), #9016, .T. ) ;
#22588=ORIENTED_EDGE ( 'NONE', *, *, #8388, .T. ) ;
#22649=ORIENTED_EDGE ( 'NONE', *, *, #8862, .F. ) ;
#22662=CARTESIAN_POINT ( 'NONE',  ( 0.1755067523729419432, 0.3028750839302634112, -0.5245950337139054787 ) ) ;
#22674=CARTESIAN_POINT ( 'NONE',  ( 0.1516263115863346334, 0.2937912646890007973, 0.3972688187320929099 ) ) ;
#22692=PLANE ( 'NONE',  #18163 ) ;
#22693=EDGE_CURVE ( 'NONE', #18758, #4773, #11553, .T. ) ;
#22697=DIRECTION ( 'NONE',  ( -0.2036417511401758251, 0.9790454724845842893, -1.198984999999999602E-16 ) ) ;
#22705=VERTEX_POINT ( 'NONE', #18316 ) ;
#22706=CARTESIAN_POINT ( 'NONE',  ( 0.3680051700917441604, 0.000000000000000000, 0.000000000000000000 ) ) ;
#22729=CARTESIAN_POINT ( 'NONE',  ( 0.5925575908939920700, 0.000000000000000000, 0.000000000000000000 ) ) ;
#22746=ORIENTED_EDGE ( 'NONE', *, *, #27831, .T. ) ;
#22779=CARTESIAN_POINT ( 'NONE',  ( 0.1516263115863346334, 0.2937912646890004087, -0.3972688187320929099 ) ) ;
#22782=CIRCLE ( 'NONE', #12865, 0.3346456692913385988 ) ;
#22799=CARTESIAN_POINT ( 'NONE',  ( 0.1506723201675407575, 0.000000000000000000, 0.000000000000000000 ) ) ;
#22807=VERTEX_POINT ( 'NONE', #27808 ) ;
#22810=ADVANCED_FACE ( 'NONE', ( #20880 ), #24954, .T. ) ;
#22816=CONICAL_SURFACE ( 'NONE', #12451, 0.1106489370078740098, 0.08726646250000029414 ) ;
#22821=DIRECTION ( 'NONE',  ( -0.9930684569432060016, -0.05876869877843096668, -0.1017903721789526900 ) ) ;
#22824=VERTEX_POINT ( 'NONE', #6062 ) ;
#22856=EDGE_CURVE ( 'NONE', #13737, #14598, #524, .T. ) ;
#22859=CONICAL_SURFACE ( 'NONE', #22400, 0.4537419570391968415, 1.365720138124999927 ) ;
#22879=DIRECTION ( 'NONE',  ( 0.2036417511401769631, -0.9790454724845838452, 1.198984999999999849E-16 ) ) ;
#22899=AXIS2_PLACEMENT_3D ( 'NONE', #4723, #3155, #13347 ) ;
#22932=CIRCLE ( 'NONE', #14375, 0.4267795243146149664 ) ;
#22936=CARTESIAN_POINT ( 'NONE',  ( 0.000000000000000000, 0.000000000000000000, 0.000000000000000000 ) ) ;
#22939=CARTESIAN_POINT ( 'NONE',  ( 0.1522836969735573143, 0.000000000000000000, 0.000000000000000000 ) ) ;
#22943=EDGE_CURVE ( 'NONE', #23305, #16322, #2815, .T. ) ;
#22946=CARTESIAN_POINT ( 'NONE',  ( 0.1522836969815822838, 0.1970374587168192970, 0.4531137400420984229 ) ) ;
#22960=ORIENTED_EDGE ( 'NONE', *, *, #18122, .F. ) ;
#22961=ORIENTED_EDGE ( 'NONE', *, *, #284, .T. ) ;
#22973=ADVANCED_FACE ( 'NONE', ( #13794 ), #22692, .T. ) ;
#23019=EDGE_LOOP ( 'NONE', ( #7086, #8778, #9674, #11666, #13065 ) ) ;
#23026=DIRECTION ( 'NONE',  ( 0.000000000000000000, 1.000000000000000000, 0.000000000000000000 ) ) ;
#23053=FILL_AREA_STYLE_COLOUR ( '', #12141 ) ;
#23061=ORIENTED_EDGE ( 'NONE', *, *, #23097, .T. ) ;
#23077=DIRECTION ( 'NONE',  ( -0.9575713608335526539, -0.2881962680386024878, 2.462036256411297774E-17 ) ) ;
#23078=DIRECTION ( 'NONE',  ( 0.000000000000000000, -1.000000000000000000, 0.000000000000000000 ) ) ;
#23097=EDGE_CURVE ( 'NONE', #15651, #25542, #12374, .T. ) ;
#23141=CARTESIAN_POINT ( 'NONE',  ( 0.03937007874015747977, 4.339299682018180063E-17, 0.3346456692913385988 ) ) ;
#23161=CONICAL_SURFACE ( 'NONE', #20890, 0.4537419570391968415, 1.365720138124999927 ) ;
#23169=AXIS2_PLACEMENT_3D ( 'NONE', #16382, #3507, #12006 ) ;
#23173=CARTESIAN_POINT ( 'NONE',  ( 0.1518453843511950729, -0.4909359254672716610, -0.05583672882996244813 ) ) ;
#23183=AXIS2_PLACEMENT_3D ( 'NONE', #11331, #27009, #13580 ) ;
#23185=ORIENTED_EDGE ( 'NONE', *, *, #4130, .F. ) ;
#23188=ORIENTED_EDGE ( 'NONE', *, *, #8343, .T. ) ;
#23196=VERTEX_POINT ( 'NONE', #1639 ) ;
#23197=( LENGTH_UNIT ( ) NAMED_UNIT ( * ) SI_UNIT ( $, .METRE. ) ) ;
#23202=CARTESIAN_POINT ( 'NONE',  ( 0.1490609433615242285, 0.2393035190771452825, -0.4144858534716441278 ) ) ;
#23215=EDGE_CURVE ( 'NONE', #15651, #22705, #1917, .T. ) ;
#23219=ORIENTED_EDGE ( 'NONE', *, *, #2597, .F. ) ;
#23234=CARTESIAN_POINT ( 'NONE',  ( 0.000000000000000000, 0.000000000000000000, 0.000000000000000000 ) ) ;
#23248=ORIENTED_EDGE ( 'NONE', *, *, #3359, .F. ) ;
#23256=DIRECTION ( 'NONE',  ( 0.000000000000000000, 1.000000000000000000, 0.000000000000000000 ) ) ;
#23260=CIRCLE ( 'NONE', #11067, 0.03937007874015744507 ) ;
#23276=CARTESIAN_POINT ( 'NONE',  ( 0.000000000000000000, 0.000000000000000000, 0.000000000000000000 ) ) ;
#23281=CARTESIAN_POINT ( 'NONE',  ( 0.1522836969735573143, -0.1970374587079582740, -0.4531137400369409374 ) ) ;
#23305=VERTEX_POINT ( 'NONE', #68 ) ;
#23317=CARTESIAN_POINT ( 'NONE',  ( 0.07614184848677874040, -0.4941010236220472751, 6.050992370341708321E-17 ) ) ;
#23322=DIRECTION ( 'NONE',  ( 0.2036417511401759084, -0.4895227362422918116, -0.8478782506317885659 ) ) ;
#23334=ORIENTED_EDGE ( 'NONE', *, *, #23097, .F. ) ;
#23339=VERTEX_POINT ( 'NONE', #2137 ) ;
#23350=PRESENTATION_STYLE_ASSIGNMENT (( #9902 ) ) ;
#23386=CARTESIAN_POINT ( 'NONE',  ( 0.1495939273659966928, 0.4806208190371651368, 0.02345246241340225024 ) ) ;
#23408=ORIENTED_EDGE ( 'NONE', *, *, #10333, .F. ) ;
#23410=LINE ( 'NONE', #8144, #14781 ) ;
#23435=ORIENTED_EDGE ( 'NONE', *, *, #1186, .T. ) ;
#23450=CARTESIAN_POINT ( 'NONE',  ( 0.5981657849660177995, -0.2403521948818897747, 0.4163022132461299263 ) ) ;
#23457=LINE ( 'NONE', #23317, #21664 ) ;
#23480=CARTESIAN_POINT ( 'NONE',  ( 0.3905379133858267737, -0.2805118110236220486, -0.4858607088160724063 ) ) ;
#23499=DIRECTION ( 'NONE',  ( -0.9575713608335526539, 0.2881962680386024878, 1.067350012615773080E-17 ) ) ;
#23538=VECTOR ( 'NONE', #19007, 39.37007874015748143 ) ;
#23568=CARTESIAN_POINT ( 'NONE',  ( 0.1522836969735573143, 0.2938892803217901806, -0.3971963147566898167 ) ) ;
#23584=CIRCLE ( 'NONE', #9558, 0.3346456692913385988 ) ;
#23594=ORIENTED_EDGE ( 'NONE', *, *, #26948, .T. ) ;
#23600=AXIS2_PLACEMENT_3D ( 'NONE', #9147, #17767, #11415 ) ;
#23611=CIRCLE ( 'NONE', #3719, 0.1298643763538142593 ) ;
#23618=EDGE_LOOP ( 'NONE', ( #15776, #24107, #1810, #22397 ) ) ;
#23653=CARTESIAN_POINT ( 'NONE',  ( 0.1490609433576163545, 0.2393035190829114200, 0.4144858534816307505 ) ) ;
#23660=EDGE_CURVE ( 'NONE', #13737, #14598, #14717, .T. ) ;
#23676=FACE_OUTER_BOUND ( 'NONE', #116, .T. ) ;
#23730=EDGE_CURVE ( 'NONE', #22824, #11643, #11430, .T. ) ;
#23735=LINE ( 'NONE', #21472, #25008 ) ;
#23771=DIRECTION ( 'NONE',  ( -1.000000000000000000, 0.000000000000000000, 0.000000000000000000 ) ) ;
#23788=B_SPLINE_CURVE_WITH_KNOTS ( 'NONE', 3,
 ( #14573, #1684, #17362, #11135, #10726, #10859 ),
 .UNSPECIFIED., .F., .F.,
 ( 4, 2, 4 ),
 ( 4.333759502428735381E-14, 0.0007294371397779527647, 0.001458874279512567800 ),
 .UNSPECIFIED. ) ;
#23815=CARTESIAN_POINT ( 'NONE',  ( 0.5869493968219645641, 0.000000000000000000, 0.000000000000000000 ) ) ;
#23841=VERTEX_POINT ( 'NONE', #11540 ) ;
#23898=DIRECTION ( 'NONE',  ( -0.2036417511401758251, 0.4895227362422921447, 0.8478782506317885659 ) ) ;
#23906=ADVANCED_FACE ( 'NONE', ( #26792 ), #7439, .T. ) ;
#23909=ORIENTED_EDGE ( 'NONE', *, *, #373, .F. ) ;
#23919=ORIENTED_EDGE ( 'NONE', *, *, #12310, .F. ) ;
#23938=CIRCLE ( 'NONE', #17185, 0.3346456692913385988 ) ;
#23965=DIRECTION ( 'NONE',  ( -0.9790454724845839563, -0.1018208755700888840, 0.1763589297585419768 ) ) ;
#23970=ORIENTED_EDGE ( 'NONE', *, *, #380, .F. ) ;
#23991=DIRECTION ( 'NONE',  ( -0.2036417511401758251, -0.9790454724845842893, 0.000000000000000000 ) ) ;
#24014=CARTESIAN_POINT ( 'NONE',  ( 0.1522836969735573143, 0.4909267390297480382, -0.05591742528025173131 ) ) ;
#24031=EDGE_CURVE ( 'NONE', #1011, #21566, #24333, .T. ) ;
#24033=VERTEX_POINT ( 'NONE', #5074 ) ;
#24049=AXIS2_PLACEMENT_3D ( 'NONE', #13159, #19938, #11456 ) ;
#24050=CARTESIAN_POINT ( 'NONE',  ( 0.5981657849660177995, 0.2403521948818897747, 0.4163022132461299263 ) ) ;
#24107=ORIENTED_EDGE ( 'NONE', *, *, #13842, .F. ) ;
#24126=DIRECTION ( 'NONE',  ( -0.1772802999855984940, 0.000000000000000000, 0.9841604011730080703 ) ) ;
#24129=CARTESIAN_POINT ( 'NONE',  ( 0.000000000000000000, 0.000000000000000000, 0.000000000000000000 ) ) ;
#24132=EDGE_CURVE ( 'NONE', #24341, #8473, #6052, .T. ) ;
#24146=( BOUNDED_CURVE ( )  B_SPLINE_CURVE ( 3, ( #11188, #2560, #468, #15176 ),
 .UNSPECIFIED., .F., .F. ) 
 B_SPLINE_CURVE_WITH_KNOTS ( ( 4, 4 ),
 ( 6.170019055269734487, 6.396351559089437089 ),
 .UNSPECIFIED. ) 
 CURVE ( )  GEOMETRIC_REPRESENTATION_ITEM ( )  RATIONAL_B_SPLINE_CURVE ( ( 1.000000000000000000, 0.9957356870045845909, 0.9957356870045845909, 1.000000000000000000 ) ) 
 REPRESENTATION_ITEM ( '' )  ) ;
#24153=DIRECTION ( 'NONE',  ( -0.9930684569549264040, -0.05876869872891801738, -0.1017903720931950112 ) ) ;
#24174=ORIENTED_EDGE ( 'NONE', *, *, #26340, .T. ) ;
#24214=CARTESIAN_POINT ( 'NONE',  ( 0.1522836969735573143, 0.1970374587079574968, -0.4531137400369417145 ) ) ;
#24261=LINE ( 'NONE', #11137, #2629 ) ;
#24295=CARTESIAN_POINT ( 'NONE',  ( 0.1520645003235147619, 0.4909313315706889669, -0.05587710509139291737 ) ) ;
#24300=DIRECTION ( 'NONE',  ( 0.000000000000000000, 1.000000000000000000, 0.000000000000000000 ) ) ;
#24308=DIRECTION ( 'NONE',  ( 0.000000000000000000, 1.000000000000000000, 0.000000000000000000 ) ) ;
#24333=B_SPLINE_CURVE_WITH_KNOTS ( 'NONE', 3,
 ( #18196, #11439, #24295, #7484 ),
 .UNSPECIFIED., .F., .F.,
 ( 4, 4 ),
 ( 1.726099910371974966, 1.727746213436275102 ),
 .UNSPECIFIED. ) ;
#24336=CARTESIAN_POINT ( 'NONE',  ( 0.6299212598425196763, 0.000000000000000000, 0.000000000000000000 ) ) ;
#24341=VERTEX_POINT ( 'NONE', #20112 ) ;
#24350=CARTESIAN_POINT ( 'NONE',  ( 0.5905511811023621549, 0.000000000000000000, 0.000000000000000000 ) ) ;
#24353=EDGE_CURVE ( 'NONE', #4182, #11023, #25039, .T. ) ;
#24366=EDGE_CURVE ( 'NONE', #15615, #16233, #22334, .T. ) ;
#24371=ORIENTED_EDGE ( 'NONE', *, *, #14585, .F. ) ;
#24396=DIRECTION ( 'NONE',  ( 0.2036417511401770464, 0.4895227362422922002, 0.8478782506317882328 ) ) ;
#24400=APPLICATION_CONTEXT ( 'automotive_design' ) ;
#24402=VECTOR ( 'NONE', #5715, 39.37007874015748854 ) ;
#24405=DIRECTION ( 'NONE',  ( 0.000000000000000000, -0.8660254037844384856, 0.5000000000000003331 ) ) ;
#24412=DIRECTION ( 'NONE',  ( 1.000000000000000000, 0.000000000000000000, 0.000000000000000000 ) ) ;
#24418=DIMENSIONAL_EXPONENTS ( 1.000000000000000000, 0.000000000000000000, 0.000000000000000000, 0.000000000000000000, 0.000000000000000000, 0.000000000000000000, 0.000000000000000000 ) ;
#24426=CARTESIAN_POINT ( 'NONE',  ( 0.5869493968219645641, 0.4267795243146149664, 0.000000000000000000 ) ) ;
#24438=ORIENTED_EDGE ( 'NONE', *, *, #24132, .T. ) ;
#24440=VERTEX_POINT ( 'NONE', #1592 ) ;
#24478=CARTESIAN_POINT ( 'NONE',  ( 0.1493295869868995762, -0.2561000767422981772, -0.4059580611872550260 ) ) ;
#24483=DIRECTION ( 'NONE',  ( -1.000000000000000000, 0.000000000000000000, 0.000000000000000000 ) ) ;
#24484=DIRECTION ( 'NONE',  ( 0.000000000000000000, 0.000000000000000000, -1.000000000000000000 ) ) ;
#24507=CARTESIAN_POINT ( 'NONE',  ( 0.1495939273659337154, 0.2606208377493157702, -0.4045036076671820746 ) ) ;
#24510=EDGE_LOOP ( 'NONE', ( #16052, #9656, #1125, #16484 ) ) ;
#24554=DIRECTION ( 'NONE',  ( -0.2036417511401762415, -0.4895227362422910344, 0.8478782506317890100 ) ) ;
#24577=EDGE_CURVE ( 'NONE', #8473, #4752, #15116, .T. ) ;
#24580=EDGE_LOOP ( 'NONE', ( #19668, #22109, #8453, #25361, #12213, #25290 ) ) ;
#24587=CIRCLE ( 'NONE', #9713, 0.4941010236220472751 ) ;
#24617=DIRECTION ( 'NONE',  ( 0.000000000000000000, 1.000000000000000000, 0.000000000000000000 ) ) ;
#24640=DIRECTION ( 'NONE',  ( -0.2036417511401758251, -0.4895227362422921447, -0.8478782506317885659 ) ) ;
#24658=DIRECTION ( 'NONE',  ( -0.9790454724845842893, -0.2036417511401760472, 2.493892000000000781E-17 ) ) ;
#24684=ORIENTED_EDGE ( 'NONE', *, *, #22320, .T. ) ;
#24697=CARTESIAN_POINT ( 'NONE',  ( 0.6299212598425196763, 0.000000000000000000, 0.000000000000000000 ) ) ;
#24764=CARTESIAN_POINT ( 'NONE',  ( 0.1522836969735573143, -0.1970374587079578854, 0.4531137400369409374 ) ) ;
#24774=AXIS2_PLACEMENT_3D ( 'NONE', #10464, #10604, #23898 ) ;
#24937=VERTEX_POINT ( 'NONE', #26500 ) ;
#24944=DIRECTION ( 'NONE',  ( 0.9930684569549264040, -0.05876869872891801738, -0.1017903720931950112 ) ) ;
#24946=DIRECTION ( 'NONE',  ( 0.000000000000000000, 0.000000000000000000, -1.000000000000000000 ) ) ;
#24954=CONICAL_SURFACE ( 'NONE', #12779, 0.4526932812344527379, 0.1178097243749990780 ) ;
#24977=ORIENTED_EDGE ( 'NONE', *, *, #3137, .T. ) ;
#24989=CARTESIAN_POINT ( 'NONE',  ( 0.1522836969735573143, -0.4909267390297480382, -0.05591742528025173131 ) ) ;
#25008=VECTOR ( 'NONE', #1832, 39.37007874015748854 ) ;
#25035=DIRECTION ( 'NONE',  ( 1.000000000000000000, 0.000000000000000000, 0.000000000000000000 ) ) ;
#25037=EDGE_CURVE ( 'NONE', #21046, #16610, #16012, .T. ) ;
#25039=B_SPLINE_CURVE_WITH_KNOTS ( 'NONE', 3,
 ( #16167, #9359, #11497, #5427, #1330, #24478, #11921, #13613 ),
 .UNSPECIFIED., .F., .F.,
 ( 4, 2, 2, 4 ),
 ( 0.000000000000000000, 0.2500000000000000000, 0.5000000000000000000, 1.000000000000000000 ),
 .UNSPECIFIED. ) ;
#25046=CARTESIAN_POINT ( 'NONE',  ( 0.3905379133858267737, -0.5610236220472440971, 6.870559055118111198E-17 ) ) ;
#25065=CIRCLE ( 'NONE', #12892, 0.4941010236220472751 ) ;
#25077=B_SPLINE_CURVE_WITH_KNOTS ( 'NONE', 3,
 ( #20585, #9838, #8293, #10821 ),
 .UNSPECIFIED., .F., .F.,
 ( 4, 4 ),
 ( 1.006307675027575899, 1.007953978091874037 ),
 .UNSPECIFIED. ) ;
#25086=CARTESIAN_POINT ( 'NONE',  ( 0.5869493968219645641, 0.2133897621573074832, -0.3696019098714952711 ) ) ;
#25092=FACE_OUTER_BOUND ( 'NONE', #20641, .T. ) ;
#25112=LINE ( 'NONE', #22575, #27771 ) ;
#25141=DIRECTION ( 'NONE',  ( 0.9930684569549264040, 0.05876869872891801738, -0.1017903720931950112 ) ) ;
#25150=CARTESIAN_POINT ( 'NONE',  ( 0.1520643344662694629, 0.4930463976998556985, 0.03726710077533022109 ) ) ;
#25168=LINE ( 'NONE', #5407, #11448 ) ;
#25181=DIRECTION ( 'NONE',  ( 0.000000000000000000, 1.000000000000000000, 0.000000000000000000 ) ) ;
#25184=CARTESIAN_POINT ( 'NONE',  ( 0.5869493968219645641, -0.2133897621573074832, 0.3696019098714952711 ) ) ;
#25189=LINE ( 'NONE', #27750, #24402 ) ;
#25191=EDGE_CURVE ( 'NONE', #12210, #22329, #14917, .T. ) ;
#25233=VECTOR ( 'NONE', #6544, 39.37007874015748143 ) ;
#25240=ADVANCED_FACE ( 'NONE', ( #14944 ), #6986, .T. ) ;
#25241=ORIENTED_EDGE ( 'NONE', *, *, #665, .T. ) ;
#25245=DIRECTION ( 'NONE',  ( -0.2036417511401759362, -0.4895227362422912565, 0.8478782506317890100 ) ) ;
#25256=DIRECTION ( 'NONE',  ( -1.000000000000000000, 0.000000000000000000, 0.000000000000000000 ) ) ;
#25265=ORIENTED_EDGE ( 'NONE', *, *, #12351, .F. ) ;
#25271=CARTESIAN_POINT ( 'NONE',  ( 0.1520645003680120011, 0.4909313315697558799, 0.05587710509957802968 ) ) ;
#25273=EDGE_CURVE ( 'NONE', #4752, #8473, #17371, .T. ) ;
#25274=AXIS2_PLACEMENT_3D ( 'NONE', #7648, #11593, #27002 ) ;
#25290=ORIENTED_EDGE ( 'NONE', *, *, #13492, .F. ) ;
#25350=EDGE_LOOP ( 'NONE', ( #4988, #7133, #5953, #27537 ) ) ;
#25352=ORIENTED_EDGE ( 'NONE', *, *, #23215, .T. ) ;
#25361=ORIENTED_EDGE ( 'NONE', *, *, #24353, .F. ) ;
#25369=CARTESIAN_POINT ( 'NONE',  ( 0.5869493968219645641, 0.2133897621573074832, -0.3696019098714952711 ) ) ;
#25389=CARTESIAN_POINT ( 'NONE',  ( 0.1491281042588007977, -0.4788599204499175421, -0.009432676026062585331 ) ) ;
#25398=ORIENTED_EDGE ( 'NONE', *, *, #11996, .F. ) ;
#25400=DIRECTION ( 'NONE',  ( 1.000000000000000000, 0.000000000000000000, 0.000000000000000000 ) ) ;
#25432=CARTESIAN_POINT ( 'NONE',  ( 0.5869493968219645641, -0.2133897621573074832, 0.3696019098714952711 ) ) ;
#25438=AXIS2_PLACEMENT_3D ( 'NONE', #2644, #20440, #24126 ) ;
#25504=CARTESIAN_POINT ( 'NONE',  ( 0.1516263115863346334, -0.2937912646890007973, 0.3972688187320929099 ) ) ;
#25542=VERTEX_POINT ( 'NONE', #23202 ) ;
#25550=FACE_OUTER_BOUND ( 'NONE', #27578, .T. ) ;
#25564=CONICAL_SURFACE ( 'NONE', #26422, 0.1106489370078739681, 0.08726646250000029414 ) ;
#25580=CIRCLE ( 'NONE', #7519, 0.4267795243146149664 ) ;
#25600=LINE ( 'NONE', #8775, #14181 ) ;
#25603=CARTESIAN_POINT ( 'NONE',  ( 0.1516263115863346334, -0.2937912646890007973, 0.3972688187320929099 ) ) ;
#25614=CONICAL_SURFACE ( 'NONE', #12524, 0.1106489370078740375, 0.08726646250000029414 ) ;
#25621=DIRECTION ( 'NONE',  ( 0.000000000000000000, 1.000000000000000000, 0.000000000000000000 ) ) ;
#25643=CARTESIAN_POINT ( 'NONE',  ( 0.1490609433615242285, 0.000000000000000000, 0.000000000000000000 ) ) ;
#25656=AXIS2_PLACEMENT_3D ( 'NONE', #1275, #16673, #7777 ) ;
#25701=CARTESIAN_POINT ( 'NONE',  ( 0.5925575908939920700, 0.2268709785195988371, 0.3929520615588121824 ) ) ;
#25736=AXIS2_PLACEMENT_3D ( 'NONE', #21099, #27749, #3715 ) ;
#25763=AXIS2_PLACEMENT_3D ( 'NONE', #18415, #15766, #7413 ) ;
#25771=EDGE_CURVE ( 'NONE', #19740, #7963, #27309, .T. ) ;
#25778=DIRECTION ( 'NONE',  ( 1.000000000000000000, 0.000000000000000000, 0.000000000000000000 ) ) ;
#25812=CARTESIAN_POINT ( 'NONE',  ( 0.1638952246732497953, -0.2749627978706437048, 0.4762495361032464958 ) ) ;
#25816=DIRECTION ( 'NONE',  ( -0.2036417511401758251, 0.4895227362422921447, 0.8478782506317885659 ) ) ;
#25861=ORIENTED_EDGE ( 'NONE', *, *, #26340, .F. ) ;
#25869=EDGE_CURVE ( 'NONE', #11023, #5524, #6099, .T. ) ;
#25887=ORIENTED_EDGE ( 'NONE', *, *, #20391, .T. ) ;
#25888=ORIENTED_EDGE ( 'NONE', *, *, #23660, .T. ) ;
#25959=DIRECTION ( 'NONE',  ( 0.000000000000000000, 1.000000000000000000, 0.000000000000000000 ) ) ;
#25968=EDGE_LOOP ( 'NONE', ( #25861, #27501 ) ) ;
#25969=ORIENTED_EDGE ( 'NONE', *, *, #20565, .T. ) ;
#25985=CIRCLE ( 'NONE', #17409, 0.4786070381542913421 ) ;
#26002=FACE_OUTER_BOUND ( 'NONE', #2420, .T. ) ;
#26056=EDGE_CURVE ( 'NONE', #19645, #1011, #6617, .T. ) ;
#26091=CARTESIAN_POINT ( 'NONE',  ( 0.1493967478962657525, 0.2562458715718933799, -0.4061682508616698550 ) ) ;
#26125=ORIENTED_EDGE ( 'NONE', *, *, #21299, .T. ) ;
#26143=DIRECTION ( 'NONE',  ( 0.000000000000000000, 1.000000000000000000, 0.000000000000000000 ) ) ;
#26145=DIRECTION ( 'NONE',  ( -0.9790454724845842893, -0.1018208755700882318, 0.1763589297585410332 ) ) ;
#26150=CARTESIAN_POINT ( 'NONE',  ( 0.6140435224042697371, 0.000000000000000000, 0.000000000000000000 ) ) ;
#26195=VECTOR ( 'NONE', #22285, 39.37007874015748854 ) ;
#26196=CARTESIAN_POINT ( 'NONE',  ( 0.1490609433615242285, 0.000000000000000000, 0.000000000000000000 ) ) ;
#26204=ADVANCED_FACE ( 'NONE', ( #17652 ), #22816, .T. ) ;
#26205=ORIENTED_EDGE ( 'NONE', *, *, #25273, .F. ) ;
#26210=ORIENTED_EDGE ( 'NONE', *, *, #27426, .T. ) ;
#26229=AXIS2_PLACEMENT_3D ( 'NONE', #22799, #21246, #19113 ) ;
#26244=EDGE_CURVE ( 'NONE', #21106, #6811, #16972, .T. ) ;
#26310=CIRCLE ( 'NONE', #23169, 0.4786070381542913421 ) ;
#26322=CYLINDRICAL_SURFACE ( 'NONE', #9263, 0.4941010236220472751 ) ;
#26340=EDGE_CURVE ( 'NONE', #24033, #20796, #13789, .T. ) ;
#26341=AXIS2_PLACEMENT_3D ( 'NONE', #26150, #15303, #16987 ) ;
#26358=ORIENTED_EDGE ( 'NONE', *, *, #21922, .F. ) ;
#26366=DIRECTION ( 'NONE',  ( 1.000000000000000000, 0.000000000000000000, 0.000000000000000000 ) ) ;
#26378=CARTESIAN_POINT ( 'NONE',  ( 0.1504778549385778763, 0.2093060460840753811, -0.4379983118630946248 ) ) ;
#26382=AXIS2_PLACEMENT_3D ( 'NONE', #12403, #3927, #5015 ) ;
#26401=CARTESIAN_POINT ( 'NONE',  ( 0.5869493968219645641, -0.2133897621573074832, 0.3696019098714952711 ) ) ;
#26422=AXIS2_PLACEMENT_3D ( 'NONE', #23480, #4110, #12710 ) ;
#26465=PLANE ( 'NONE',  #1933 ) ;
#26469=B_SPLINE_CURVE_WITH_KNOTS ( 'NONE', 3,
 ( #15928, #11683, #679, #26378, #7038, #26506, #13810, #2773 ),
 .UNSPECIFIED., .F., .F.,
 ( 4, 2, 2, 4 ),
 ( 0.000000000000000000, 0.2500000000000009437, 0.5000000000000018874, 1.000000000000000000 ),
 .UNSPECIFIED. ) ;
#26476=ORIENTED_EDGE ( 'NONE', *, *, #13492, .T. ) ;
#26479=LINE ( 'NONE', #5148, #16766 ) ;
#26500=CARTESIAN_POINT ( 'NONE',  ( 0.1522836969735573143, 0.4909267390297480382, 0.05591742528025173131 ) ) ;
#26502=VECTOR ( 'NONE', #8107, 39.37007874015748143 ) ;
#26506=CARTESIAN_POINT ( 'NONE',  ( 0.1493295869868995207, 0.2235199554877277395, -0.4247682029637843693 ) ) ;
#26551=EDGE_CURVE ( 'NONE', #23339, #19765, #9316, .T. ) ;
#26552=AXIS2_PLACEMENT_3D ( 'NONE', #12798, #19150, #21285 ) ;
#26570=AXIS2_PLACEMENT_3D ( 'NONE', #11697, #16230, #13824 ) ;
#26584=EDGE_CURVE ( 'NONE', #16610, #21046, #20096, .T. ) ;
#26589=( NAMED_UNIT ( * ) SI_UNIT ( $, .STERADIAN. ) SOLID_ANGLE_UNIT ( ) ) ;
#26610=CARTESIAN_POINT ( 'NONE',  ( 0.1490609433576163545, 0.2393035190829114200, 0.4144858534816307505 ) ) ;
#26628=CARTESIAN_POINT ( 'NONE',  ( 0.1491281042588008532, 0.2475988972899728913, -0.4099885179503245936 ) ) ;
#26651=CARTESIAN_POINT ( 'NONE',  ( 0.1522836969735573143, -0.2938892803217901806, -0.3971963147566889840 ) ) ;
#26666=CONICAL_SURFACE ( 'NONE', #9065, 0.1106489370078740375, 0.08726646250000029414 ) ;
#26676=CARTESIAN_POINT ( 'NONE',  ( 0.1504778549386419362, 0.4839706879304455089, -0.03773480285758093467 ) ) ;
#26682=EDGE_CURVE ( 'NONE', #24033, #12691, #10645, .T. ) ;
#26691=DIRECTION ( 'NONE',  ( -1.000000000000000000, 0.000000000000000000, 0.000000000000000000 ) ) ;
#26776=EDGE_LOOP ( 'NONE', ( #20834, #14060, #7572, #23408, #2072, #9926 ) ) ;
#26779=ORIENTED_EDGE ( 'NONE', *, *, #26551, .F. ) ;
#26792=FACE_OUTER_BOUND ( 'NONE', #2068, .T. ) ;
#26797=VERTEX_POINT ( 'NONE', #10031 ) ;
#26801=DIRECTION ( 'NONE',  ( -0.9790454724845842893, 0.2036417511401760472, 0.000000000000000000 ) ) ;
#26827=DIRECTION ( 'NONE',  ( -0.2036417511401758251, 0.4895227362422921447, -0.8478782506317885659 ) ) ;
#26838=AXIS2_PLACEMENT_3D ( 'NONE', #27084, #24658, #22697 ) ;
#26920=ADVANCED_FACE ( 'NONE', ( #16965 ), #25564, .T. ) ;
#26938=DIRECTION ( 'NONE',  ( -0.9790454724845842893, -0.2036417511401760472, 2.493892000000000781E-17 ) ) ;
#26941=CARTESIAN_POINT ( 'NONE',  ( 0.5925575908939920700, 0.4537419570391968415, 0.000000000000000000 ) ) ;
#26948=EDGE_CURVE ( 'NONE', #12947, #4526, #22298, .T. ) ;
#26975=CARTESIAN_POINT ( 'NONE',  ( 0.1518453843511950729, 0.4909359254672716610, 0.05583672882996252446 ) ) ;
#26980=VERTEX_POINT ( 'NONE', #8889 ) ;
#26987=LINE ( 'NONE', #16115, #27285 ) ;
#26990=CIRCLE ( 'NONE', #12561, 0.4807043897637795493 ) ;
#27002=DIRECTION ( 'NONE',  ( 0.000000000000000000, 1.000000000000000000, 0.000000000000000000 ) ) ;
#27009=DIRECTION ( 'NONE',  ( 1.000000000000000000, 0.000000000000000000, 0.000000000000000000 ) ) ;
#27026=AXIS2_PLACEMENT_3D ( 'NONE', #24129, #546, #9141 ) ;
#27047=DIRECTION ( 'NONE',  ( -0.9790454724845842893, 0.1018208755700880375, -0.1763589297585410332 ) ) ;
#27084=CARTESIAN_POINT ( 'NONE',  ( 0.6055690743987126590, -0.5162970762339605946, 6.322814960629921339E-17 ) ) ;
#27086=CIRCLE ( 'NONE', #25736, 0.4267795243146149664 ) ;
#27089=EDGE_CURVE ( 'NONE', #14598, #22705, #3402, .T. ) ;
#27091=ORIENTED_EDGE ( 'NONE', *, *, #27427, .T. ) ;
#27102=VERTEX_POINT ( 'NONE', #17895 ) ;
#27138=ORIENTED_EDGE ( 'NONE', *, *, #26056, .F. ) ;
#27147=DIRECTION ( 'NONE',  ( 0.000000000000000000, 1.000000000000000000, 0.000000000000000000 ) ) ;
#27180=ORIENTED_EDGE ( 'NONE', *, *, #12351, .T. ) ;
#27185=DIRECTION ( 'NONE',  ( 0.9790454724845839563, 0.1018208755700887314, -0.1763589297585421989 ) ) ;
#27193=CARTESIAN_POINT ( 'NONE',  ( 0.1490609433494345937, 0.4786070381568061638, 0.004730797288071140853 ) ) ;
#27198=ADVANCED_FACE ( 'NONE', ( #25550 ), #22859, .T. ) ;
#27217=EDGE_CURVE ( 'NONE', #1802, #26980, #18112, .T. ) ;
#27224=CONICAL_SURFACE ( 'NONE', #20910, 0.4537419570391968415, 1.365720138124999927 ) ;
#27233=AXIS2_PLACEMENT_3D ( 'NONE', #13250, #17491, #23991 ) ;
#27241=CARTESIAN_POINT ( 'NONE',  ( 0.5905511811023621549, 4.580371886574746102E-17, 0.3740157480314960647 ) ) ;
#27242=ORIENTED_EDGE ( 'NONE', *, *, #9660, .F. ) ;
#27245=CARTESIAN_POINT ( 'NONE',  ( 0.1493295869868995207, -0.4796200322302701657, 0.01881014177837847870 ) ) ;
#27252=EDGE_CURVE ( 'NONE', #7492, #22807, #23410, .T. ) ;
#27283=DIRECTION ( 'NONE',  ( 1.000000000000000000, 0.000000000000000000, 0.000000000000000000 ) ) ;
#27285=VECTOR ( 'NONE', #25141, 39.37007874015748854 ) ;
#27309=CIRCLE ( 'NONE', #18265, 0.4786070381542913421 ) ;
#27321=CARTESIAN_POINT ( 'NONE',  ( 0.1490609433576163545, 0.2393035190829114200, 0.4144858534816307505 ) ) ;
#27326=CARTESIAN_POINT ( 'NONE',  ( 0.1520643344662694629, 0.4930463976998556985, -0.03726710077533019333 ) ) ;
#27327=CARTESIAN_POINT ( 'NONE',  ( 0.1522836969735573143, 0.4909267390297480382, 0.05591742528025173131 ) ) ;
#27362=CARTESIAN_POINT ( 'NONE',  ( 0.1516263115863346334, 0.1971492568089275588, 0.4530651079966787620 ) ) ;
#27412=CARTESIAN_POINT ( 'NONE',  ( 0.1522836969815822838, -0.2938892803218252081, 0.3971963147669425598 ) ) ;
#27414=AXIS2_PLACEMENT_3D ( 'NONE', #15488, #13909, #7130 ) ;
#27422=EDGE_LOOP ( 'NONE', ( #14664, #11762, #18381, #12557 ) ) ;
#27426=EDGE_CURVE ( 'NONE', #13098, #15615, #304, .T. ) ;
#27427=EDGE_CURVE ( 'NONE', #12947, #280, #25580, .T. ) ;
#27439=VECTOR ( 'NONE', #19063, 39.37007874015748143 ) ;
#27445=CIRCLE ( 'NONE', #15287, 0.1298643763538141760 ) ;
#27492=EDGE_LOOP ( 'NONE', ( #23061, #13720, #10704, #15778 ) ) ;
#27501=ORIENTED_EDGE ( 'NONE', *, *, #15964, .F. ) ;
#27537=ORIENTED_EDGE ( 'NONE', *, *, #12030, .F. ) ;
#27571=( NAMED_UNIT ( * ) PLANE_ANGLE_UNIT ( ) SI_UNIT ( $, .RADIAN. ) ) ;
#27578=EDGE_LOOP ( 'NONE', ( #20743, #25241, #23594, #17646 ) ) ;
#27584=CARTESIAN_POINT ( 'NONE',  ( 0.1755067523729419432, -0.3028750839302637998, -0.5245950337139047015 ) ) ;
#27711=DIRECTION ( 'NONE',  ( -1.000000000000000000, 0.000000000000000000, 0.000000000000000000 ) ) ;
#27717=ADVANCED_FACE ( 'NONE', ( #9747, #14544 ), #19026, .T. ) ;
#27728=DIRECTION ( 'NONE',  ( 1.000000000000000000, 0.000000000000000000, 0.000000000000000000 ) ) ;
#27749=DIRECTION ( 'NONE',  ( 1.000000000000000000, 0.000000000000000000, 0.000000000000000000 ) ) ;
#27750=CARTESIAN_POINT ( 'NONE',  ( 0.5869493968219645641, -0.4267795243146149664, 5.226543307086613929E-17 ) ) ;
#27771=VECTOR ( 'NONE', #14101, 39.37007874015748854 ) ;
#27774=ORIENTED_EDGE ( 'NONE', *, *, #3964, .T. ) ;
#27808=CARTESIAN_POINT ( 'NONE',  ( 0.5869493968219645641, -0.2133897621573074832, 0.3696019098714952711 ) ) ;
#27831=EDGE_CURVE ( 'NONE', #2655, #27102, #12024, .T. ) ;
#27842=ORIENTED_EDGE ( 'NONE', *, *, #14054, .T. ) ;
#27951=CARTESIAN_POINT ( '', ( 0.0, 0.0, 0.0 ) ) ;
#27952=DIRECTION ( '', ( 0.0, 0.0, 1.0 ) ) ;
#27953=DIRECTION ( '', ( 1.0, 0.0, 0.0 ) ) ;
#27954=AXIS2_PLACEMENT_3D ( '', #27951, #27952, #27953 ) ;
#27955=ADVANCED_BREP_SHAPE_REPRESENTATION ( 'Bearing Cone', ( #21416, #27954, #27965 ), #3496 ) ;
#27956=PRODUCT ( 'Bearing Cone', 'Bearing Cone', '', ( #7554 ) ) ;
#27957=PRODUCT_DEFINITION_FORMATION_WITH_SPECIFIED_SOURCE ( 'ANY', '', #27956, .NOT_KNOWN. ) ;
#27958=PRODUCT_DEFINITION ( 'Bearing Cone', '', #27957, #20403 ) ;
#27959=PRODUCT_DEFINITION_SHAPE ( '', '', #27958 ) ;
#27960=SHAPE_DEFINITION_REPRESENTATION ( #27959, #27955 ) ;
#27962=CARTESIAN_POINT ( '', ( 0.0, 0.0, 0.0 ) ) ;
#27963=DIRECTION ( '', ( 0.0, 0.0, 1.0 ) ) ;
#27964=DIRECTION ( '', ( 1.0, 0.0, 0.0 ) ) ;
#27965=AXIS2_PLACEMENT_3D ( '', #27962, #27963, #27964 ) ;
ENDSEC;
END-ISO-10303-21;
